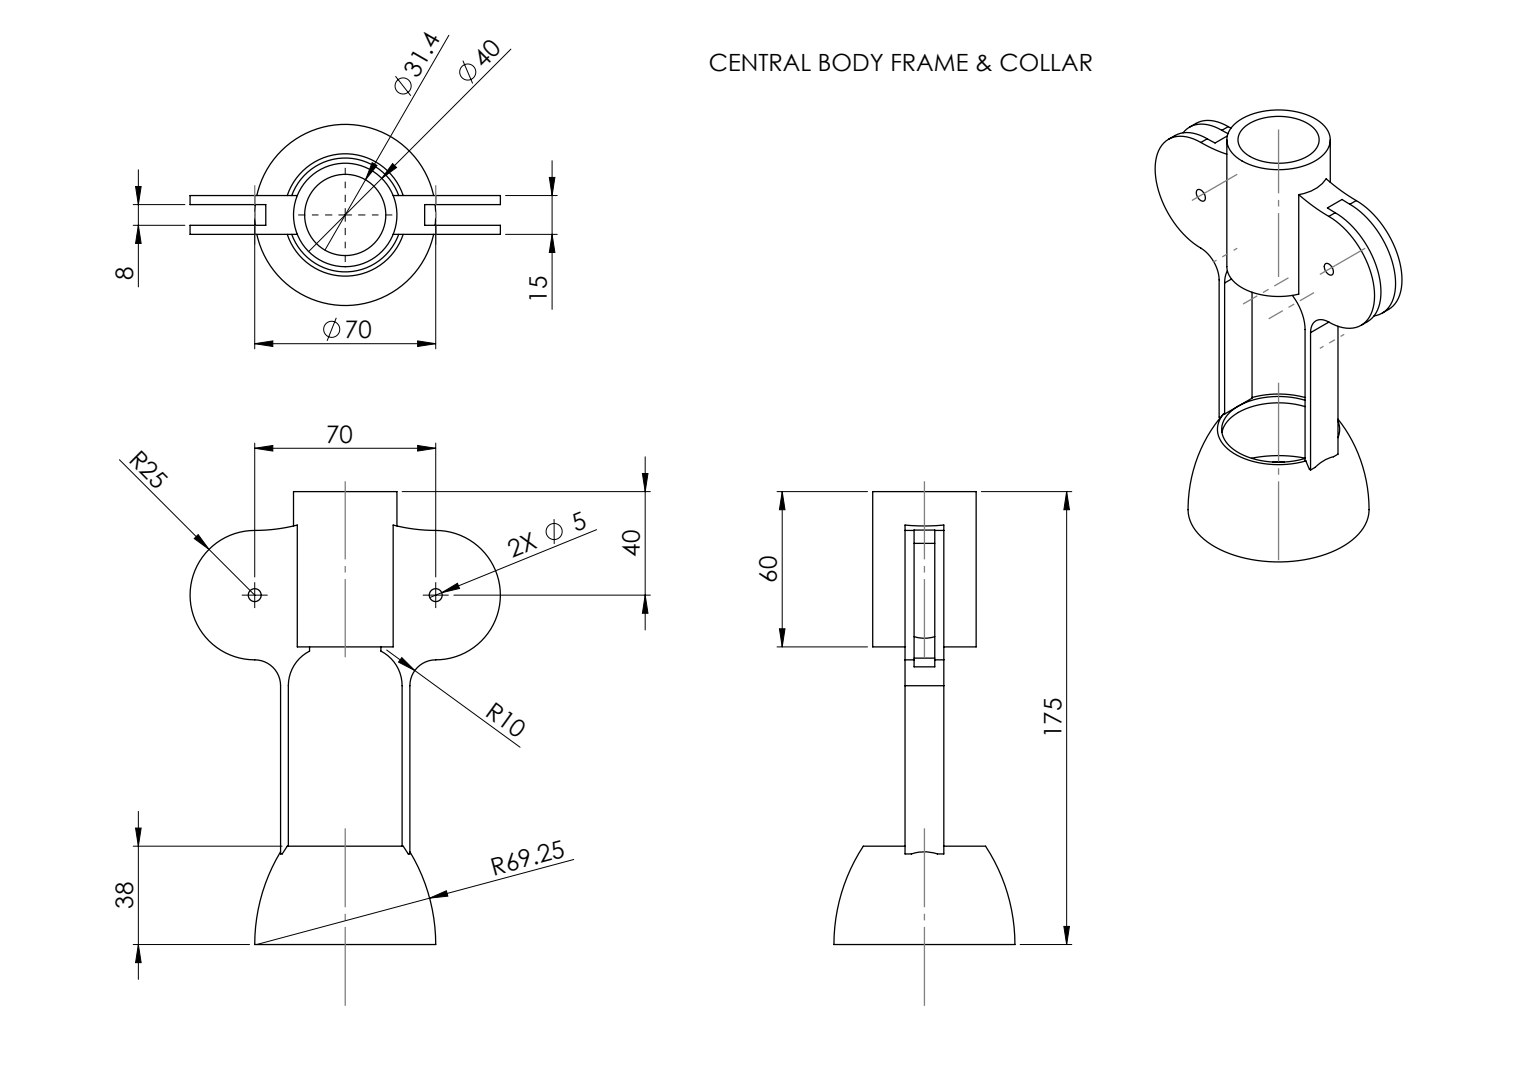
ISO-10303-21;
HEADER;
FILE_DESCRIPTION (('STEP AP214'),
    '1' );
FILE_NAME ('Central Body Frame & Collar.step',
    '2026-10-08T14:03:35',
    ( '' ),
    ( '' ),
    'SwSTEP 2.0',
    'SolidWorks 2026',
    '' );
FILE_SCHEMA (( 'AUTOMOTIVE_DESIGN' ));
ENDSEC;

DATA;
#1=EDGE_LOOP ( 'NONE', ( #6943, #8347, #5492, #144, #24, #10049, #6379, #1001, #2175, #10989 ) ) ;
#8=ORIENTED_EDGE ( 'NONE', *, *, #7820, .F. ) ;
#14=DIRECTION ( 'NONE',  ( -1.000000000000000000, 0.000000000000000000, 0.000000000000000000 ) ) ;
#18=VECTOR ( 'NONE', #6174, 1000.000000000000000 ) ;
#22=ORIENTED_EDGE ( 'NONE', *, *, #10210, .T. ) ;
#24=ORIENTED_EDGE ( 'NONE', *, *, #1458, .F. ) ;
#28=DIRECTION ( 'NONE',  ( -0.000000000000000000, -0.000000000000000000, -1.000000000000000000 ) ) ;
#33=CIRCLE ( 'NONE', #4726, 10.00000000000000178 ) ;
#35=CIRCLE ( 'NONE', #10337, 25.00000000000000711 ) ;
#39=DIRECTION ( 'NONE',  ( 1.000000000000000000, 0.000000000000000000, 0.000000000000000000 ) ) ;
#47=EDGE_LOOP ( 'NONE', ( #4618, #2570, #12122, #10874, #7639, #5291, #7255 ) ) ;
#54=CIRCLE ( 'NONE', #4755, 69.24999999999975842 ) ;
#60=DIRECTION ( 'NONE',  ( -1.000000000000000000, 0.000000000000000000, 0.000000000000000000 ) ) ;
#61=EDGE_CURVE ( 'NONE', #7055, #3214, #4012, .T. ) ;
#65=LINE ( 'NONE', #1951, #2569 ) ;
#67=CARTESIAN_POINT ( 'NONE',  ( -15.18222645069203125, -100.0000000000000000, -4.000000000000000000 ) ) ;
#69=ORIENTED_EDGE ( 'NONE', *, *, #3097, .T. ) ;
#74=ORIENTED_EDGE ( 'NONE', *, *, #8494, .F. ) ;
#75=CARTESIAN_POINT ( 'NONE',  ( -34.99999999999999289, -97.00000000000000000, -7.500000000000000000 ) ) ;
#82=CARTESIAN_POINT ( 'NONE',  ( 25.00000000000001776, -100.0000000000000000, -5.046127144242417373 ) ) ;
#91=ORIENTED_EDGE ( 'NONE', *, *, #2062, .T. ) ;
#97=CARTESIAN_POINT ( 'NONE',  ( -26.79177319725820894, -26.24642857144861807, -4.000000000000000000 ) ) ;
#98=CARTESIAN_POINT ( 'NONE',  ( -60.00000000000001421, -4.286263797015736496E-15, 7.500000000000000000 ) ) ;
#104=CARTESIAN_POINT ( 'NONE',  ( 35.00000000000000000, 4.286263797015736496E-15, 7.500000000000000000 ) ) ;
#107=ORIENTED_EDGE ( 'NONE', *, *, #7623, .T. ) ;
#113=LINE ( 'NONE', #13095, #3464 ) ;
#122=EDGE_CURVE ( 'NONE', #8713, #9553, #6328, .T. ) ;
#123=CARTESIAN_POINT ( 'NONE',  ( 35.00000000000009237, 91.25000000000046896, 4.000000000000000000 ) ) ;
#129=CARTESIAN_POINT ( 'NONE',  ( -35.00000000000000000, -4.286263797015736496E-15, 4.000000000000000000 ) ) ;
#133=EDGE_CURVE ( 'NONE', #3737, #3625, #5810, .T. ) ;
#134=ADVANCED_FACE ( 'NONE', ( #1030, #12741 ), #7261, .F. ) ;
#141=VECTOR ( 'NONE', #5529, 1000.000000000000000 ) ;
#142=CARTESIAN_POINT ( 'NONE',  ( -35.00000000000000000, 25.00000000000000000, -4.000000000000000000 ) ) ;
#144=ORIENTED_EDGE ( 'NONE', *, *, #11064, .F. ) ;
#162=ORIENTED_EDGE ( 'NONE', *, *, #8775, .F. ) ;
#165=FACE_OUTER_BOUND ( 'NONE', #5586, .T. ) ;
#171=DIRECTION ( 'NONE',  ( 0.000000000000000000, 0.000000000000000000, 1.000000000000000000 ) ) ;
#174=CYLINDRICAL_SURFACE ( 'NONE', #4487, 2.500000000000002220 ) ;
#181=DIRECTION ( 'NONE',  ( -0.000000000000000000, -0.000000000000000000, -1.000000000000000000 ) ) ;
#184=CARTESIAN_POINT ( 'NONE',  ( -35.00000000000012079, 91.25000000000045475, -7.500000000000000000 ) ) ;
#194=CARTESIAN_POINT ( 'NONE',  ( 35.00000000000000000, 4.286263797015736496E-15, 4.000000000000000000 ) ) ;
#199=AXIS2_PLACEMENT_3D ( 'NONE', #10505, #5245, #13714 ) ;
#201=AXIS2_PLACEMENT_3D ( 'NONE', #5042, #6172, #12757 ) ;
#202=ORIENTED_EDGE ( 'NONE', *, *, #10624, .T. ) ;
#208=DIRECTION ( 'NONE',  ( 1.000000000000000000, 0.000000000000000000, -0.000000000000000000 ) ) ;
#212=CARTESIAN_POINT ( 'NONE',  ( -13.79311422413708499, -100.0000000000000000, 7.500000000000000000 ) ) ;
#227=AXIS2_PLACEMENT_3D ( 'NONE', #6286, #961, #5222 ) ;
#230=ORIENTED_EDGE ( 'NONE', *, *, #3262, .F. ) ;
#231=DIRECTION ( 'NONE',  ( -1.224646799147353207E-16, 1.000000000000000000, 0.000000000000000000 ) ) ;
#234=DIRECTION ( 'NONE',  ( -1.000000000000000000, 0.000000000000000000, 0.000000000000000000 ) ) ;
#240=CARTESIAN_POINT ( 'NONE',  ( 18.54049621773915746, -20.00000000000000000, -7.500000000000000000 ) ) ;
#249=DIRECTION ( 'NONE',  ( 0.000000000000000000, -1.000000000000000000, 0.000000000000000000 ) ) ;
#253=ORIENTED_EDGE ( 'NONE', *, *, #309, .F. ) ;
#260=DIRECTION ( 'NONE',  ( 0.000000000000000000, 0.000000000000000000, 1.000000000000000000 ) ) ;
#261=FACE_OUTER_BOUND ( 'NONE', #11503, .T. ) ;
#265=ORIENTED_EDGE ( 'NONE', *, *, #867, .T. ) ;
#266=ORIENTED_EDGE ( 'NONE', *, *, #11663, .F. ) ;
#269=EDGE_CURVE ( 'NONE', #10258, #13109, #10073, .T. ) ;
#270=PRODUCT_CONTEXT ( 'NONE', #3147, 'mechanical' ) ;
#276=ADVANCED_FACE ( 'NONE', ( #3756, #3111 ), #953, .F. ) ;
#277=DIRECTION ( 'NONE',  ( -1.000000000000000000, 0.000000000000000000, 0.000000000000000000 ) ) ;
#280=AXIS2_PLACEMENT_3D ( 'NONE', #8444, #12670, #13811 ) ;
#301=EDGE_CURVE ( 'NONE', #2246, #7494, #13812, .T. ) ;
#309=EDGE_CURVE ( 'NONE', #10920, #8708, #4021, .T. ) ;
#324=ORIENTED_EDGE ( 'NONE', *, *, #2209, .F. ) ;
#325=CARTESIAN_POINT ( 'NONE',  ( -22.42156014662057473, -97.00000000000000000, -7.500000000000000000 ) ) ;
#327=CARTESIAN_POINT ( 'NONE',  ( 13.79311422413708499, -20.00000000000000355, 7.500000000000000000 ) ) ;
#328=AXIS2_PLACEMENT_3D ( 'NONE', #13578, #6044, #1960 ) ;
#332=CARTESIAN_POINT ( 'NONE',  ( -19.99988111993867079, 26.72048013816596779, 0.6453928856983819351 ) ) ;
#333=CARTESIAN_POINT ( 'NONE',  ( -35.00000000000000000, -4.286263797015736496E-15, 7.500000000000000000 ) ) ;
#340=ORIENTED_EDGE ( 'NONE', *, *, #4739, .T. ) ;
#345=DIRECTION ( 'NONE',  ( -0.000000000000000000, -0.000000000000000000, -1.000000000000000000 ) ) ;
#348=CARTESIAN_POINT ( 'NONE',  ( -37.50000000000000711, -4.286263797015736496E-15, 7.500000000000000000 ) ) ;
#360=MECHANICAL_DESIGN_GEOMETRIC_PRESENTATION_REPRESENTATION('',(#8623),#10638);
#364=CARTESIAN_POINT ( 'NONE',  ( 19.96844336951937748, 26.72776445485856911, -1.294012040295340782 ) ) ;
#373=ADVANCED_FACE ( 'NONE', ( #13878 ), #5017, .F. ) ;
#376=ORIENTED_EDGE ( 'NONE', *, *, #1897, .T. ) ;
#382=DIRECTION ( 'NONE',  ( 1.000000000000000000, 0.000000000000000000, 0.000000000000000000 ) ) ;
#396=DIRECTION ( 'NONE',  ( -0.000000000000000000, -1.000000000000000000, -0.000000000000000000 ) ) ;
#399=CARTESIAN_POINT ( 'NONE',  ( -13.79311422413708499, -21.62638421600851046, -7.500000000000000000 ) ) ;
#421=LINE ( 'NONE', #1380, #11465 ) ;
#426=FILL_AREA_STYLE ('',( #13278 ) ) ;
#432=ADVANCED_FACE ( 'NONE', ( #819 ), #1931, .T. ) ;
#433=DIRECTION ( 'NONE',  ( -1.000000000000000000, -1.224646799147353207E-16, 0.000000000000000000 ) ) ;
#450=DIRECTION ( 'NONE',  ( -0.000000000000000000, 0.000000000000000000, -1.000000000000000000 ) ) ;
#452=EDGE_CURVE ( 'NONE', #1107, #10314, #12672, .T. ) ;
#457=FACE_OUTER_BOUND ( 'NONE', #1, .T. ) ;
#463=ORIENTED_EDGE ( 'NONE', *, *, #1893, .F. ) ;
#465=CARTESIAN_POINT ( 'NONE',  ( 24.37649275748779232, -100.0000000000000000, -7.500000000000000000 ) ) ;
#466=AXIS2_PLACEMENT_3D ( 'NONE', #1579, #9018, #13326 ) ;
#470=VERTEX_POINT ( 'NONE', #11938 ) ;
#472=VECTOR ( 'NONE', #11869, 1000.000000000000000 ) ;
#473=VECTOR ( 'NONE', #3861, 1000.000000000000000 ) ;
#496=AXIS2_PLACEMENT_3D ( 'NONE', #1680, #5966, #3555 ) ;
#509=DIRECTION ( 'NONE',  ( -1.224646799147353207E-16, 1.000000000000000000, -0.000000000000000000 ) ) ;
#510=CARTESIAN_POINT ( 'NONE',  ( -35.00000000000000000, -20.00000000000000000, 7.500000000000000000 ) ) ;
#521=DIRECTION ( 'NONE',  ( 0.000000000000000000, 0.000000000000000000, 1.000000000000000000 ) ) ;
#524=CARTESIAN_POINT ( 'NONE',  ( -22.00000000000000000, -35.00000000000000000, 7.500000000000000000 ) ) ;
#535=CARTESIAN_POINT ( 'NONE',  ( 18.54049621773915746, -20.00000000000000000, -7.500000000000000000 ) ) ;
#536=ORIENTED_EDGE ( 'NONE', *, *, #1893, .T. ) ;
#540=EDGE_CURVE ( 'NONE', #2953, #6457, #12760, .T. ) ;
#543=EDGE_CURVE ( 'NONE', #5663, #11307, #11801, .T. ) ;
#548=CARTESIAN_POINT ( 'NONE',  ( 35.00000000000000711, -25.00000000000000000, 7.500000000000000000 ) ) ;
#552=CARTESIAN_POINT ( 'NONE',  ( -19.36040733361899768, 26.87219970003945591, -5.058700639371027208 ) ) ;
#557=ORIENTED_EDGE ( 'NONE', *, *, #6920, .T. ) ;
#568=AXIS2_PLACEMENT_3D ( 'NONE', #1899, #1829, #13782 ) ;
#573=EDGE_CURVE ( 'NONE', #11806, #2481, #9618, .T. ) ;
#581=CARTESIAN_POINT ( 'NONE',  ( 19.75162188639114902, 26.77857048203552992, -3.206191164072788702 ) ) ;
#595=DIRECTION ( 'NONE',  ( -1.224646799147353207E-16, 1.000000000000000000, -0.000000000000000000 ) ) ;
#597=CARTESIAN_POINT ( 'NONE',  ( 1.224646799147353217E-14, -100.0000000000000000, 0.000000000000000000 ) ) ;
#598=AXIS2_PLACEMENT_3D ( 'NONE', #9274, #3873, #2045 ) ;
#600=ORIENTED_EDGE ( 'NONE', *, *, #540, .F. ) ;
#604=VECTOR ( 'NONE', #12351, 1000.000000000000000 ) ;
#605=DIRECTION ( 'NONE',  ( 0.000000000000000000, 0.000000000000000000, 1.000000000000000000 ) ) ;
#607=ORIENTED_EDGE ( 'NONE', *, *, #7807, .T. ) ;
#613=FACE_OUTER_BOUND ( 'NONE', #10515, .T. ) ;
#618=VERTEX_POINT ( 'NONE', #399 ) ;
#626=FACE_OUTER_BOUND ( 'NONE', #13070, .T. ) ;
#628=EDGE_CURVE ( 'NONE', #12494, #2284, #10129, .T. ) ;
#635=ADVANCED_FACE ( 'NONE', ( #5923, #12382 ), #2768, .F. ) ;
#640=CARTESIAN_POINT ( 'NONE',  ( -34.99999999999999289, -135.0000000000000000, 0.000000000000000000 ) ) ;
#652=ORIENTED_EDGE ( 'NONE', *, *, #5322, .F. ) ;
#659=ORIENTED_EDGE ( 'NONE', *, *, #7380, .T. ) ;
#661=ORIENTED_EDGE ( 'NONE', *, *, #10607, .F. ) ;
#665=ORIENTED_EDGE ( 'NONE', *, *, #2832, .F. ) ;
#681=AXIS2_PLACEMENT_3D ( 'NONE', #12169, #3822, #11262 ) ;
#685=ORIENTED_EDGE ( 'NONE', *, *, #12001, .T. ) ;
#690=CARTESIAN_POINT ( 'NONE',  ( 0.000000000000000000, 0.000000000000000000, 0.000000000000000000 ) ) ;
#697=VECTOR ( 'NONE', #5522, 1000.000000000000000 ) ;
#709=CARTESIAN_POINT ( 'NONE',  ( -25.00000000000000000, -35.00000000000000000, 7.500000000000000000 ) ) ;
#711=DIRECTION ( 'NONE',  ( 0.000000000000000000, 1.000000000000000000, 0.000000000000000000 ) ) ;
#716=ORIENTED_EDGE ( 'NONE', *, *, #10582, .F. ) ;
#719=EDGE_CURVE ( 'NONE', #13879, #9113, #9755, .T. ) ;
#728=CARTESIAN_POINT ( 'NONE',  ( -14.41066181492265308, -21.94006687227777874, -6.364279405527200062 ) ) ;
#733=EDGE_LOOP ( 'NONE', ( #2396, #11229, #1811, #8877, #4164, #2069 ) ) ;
#737=VECTOR ( 'NONE', #6051, 1000.000000000000000 ) ;
#742=CARTESIAN_POINT ( 'NONE',  ( -35.00000000000000000, -4.286263797015736496E-15, -4.000000000000000000 ) ) ;
#764=CARTESIAN_POINT ( 'NONE',  ( -35.00000000000000711, -25.00000000000000711, 4.000000000000000000 ) ) ;
#766=VECTOR ( 'NONE', #12559, 1000.000000000000000 ) ;
#767=ORIENTED_EDGE ( 'NONE', *, *, #13181, .F. ) ;
#774=LINE ( 'NONE', #6035, #604 ) ;
#777=CARTESIAN_POINT ( 'NONE',  ( -35.00000000000000000, -35.00000000000000000, -7.500000000000000000 ) ) ;
#792=EDGE_CURVE ( 'NONE', #6662, #8229, #1784, .T. ) ;
#799=AXIS2_PLACEMENT_3D ( 'NONE', #2482, #11030, #5781 ) ;
#801=EDGE_CURVE ( 'NONE', #3433, #1175, #9060, .T. ) ;
#806=CARTESIAN_POINT ( 'NONE',  ( 37.50000000000000711, 4.592425496802575156E-15, 7.500000000000000000 ) ) ;
#809=DIRECTION ( 'NONE',  ( -1.224646799147353207E-16, -1.499759782661857608E-32, 1.000000000000000000 ) ) ;
#812=AXIS2_PLACEMENT_3D ( 'NONE', #11782, #8689, #9817 ) ;
#819=FACE_OUTER_BOUND ( 'NONE', #8492, .T. ) ;
#827=FACE_OUTER_BOUND ( 'NONE', #12015, .T. ) ;
#836=ORIENTED_EDGE ( 'NONE', *, *, #122, .F. ) ;
#841=LINE ( 'NONE', #11493, #7119 ) ;
#847=ORIENTED_EDGE ( 'NONE', *, *, #3025, .F. ) ;
#866=AXIS2_PLACEMENT_3D ( 'NONE', #6033, #509, #433 ) ;
#867=EDGE_CURVE ( 'NONE', #11483, #10241, #6721, .T. ) ;
#871=CARTESIAN_POINT ( 'NONE',  ( -25.00000000000000000, -35.00000000000000000, -7.500000000000000000 ) ) ;
#877=DIRECTION ( 'NONE',  ( 1.000000000000000000, 0.000000000000000000, 0.000000000000000000 ) ) ;
#896=VECTOR ( 'NONE', #3103, 1000.000000000000000 ) ;
#898=AXIS2_PLACEMENT_3D ( 'NONE', #3051, #9567, #7189 ) ;
#903=CARTESIAN_POINT ( 'NONE',  ( 32.50000000000000000, 4.286263797015736496E-15, -7.500000000000000000 ) ) ;
#907=DIRECTION ( 'NONE',  ( 0.000000000000000000, 0.000000000000000000, 1.000000000000000000 ) ) ;
#914=EDGE_LOOP ( 'NONE', ( #376, #7478 ) ) ;
#915=CIRCLE ( 'NONE', #1137, 31.93204061526060755 ) ;
#916=DIRECTION ( 'NONE',  ( -1.000000000000000000, 0.000000000000000000, 0.000000000000000000 ) ) ;
#919=B_SPLINE_CURVE_WITH_KNOTS ( 'NONE', 3,
 ( #9871, #5582, #12906, #4525, #4389, #3338, #10902, #2151 ),
 .UNSPECIFIED., .F., .F.,
 ( 4, 2, 2, 4 ),
 ( 0.02189346042269462930, 0.02442701477284300177, 0.02569379194791718973, 0.02696056912299137770 ),
 .UNSPECIFIED. ) ;
#927=CIRCLE ( 'NONE', #10546, 21.99999999999999289 ) ;
#932=CARTESIAN_POINT ( 'NONE',  ( 1.653273178848927024E-14, -135.0000000000000000, 0.000000000000000000 ) ) ;
#934=EDGE_LOOP ( 'NONE', ( #5830, #10072 ) ) ;
#939=DIRECTION ( 'NONE',  ( 1.000000000000000000, 0.000000000000000000, 0.000000000000000000 ) ) ;
#948=DIRECTION ( 'NONE',  ( -1.000000000000000000, 0.000000000000000000, 0.000000000000000000 ) ) ;
#953=PLANE ( 'NONE',  #898 ) ;
#961=DIRECTION ( 'NONE',  ( -0.000000000000000000, 0.000000000000000000, -1.000000000000000000 ) ) ;
#966=EDGE_CURVE ( 'NONE', #3769, #3176, #4398, .T. ) ;
#975=DIRECTION ( 'NONE',  ( 1.000000000000000000, 1.224646799147353207E-16, 0.000000000000000000 ) ) ;
#979=EDGE_CURVE ( 'NONE', #4467, #10258, #13122, .T. ) ;
#985=FACE_OUTER_BOUND ( 'NONE', #11435, .T. ) ;
#986=ORIENTED_EDGE ( 'NONE', *, *, #8544, .T. ) ;
#998=DIRECTION ( 'NONE',  ( -1.000000000000000000, 0.000000000000000000, 0.000000000000000000 ) ) ;
#1000=ORIENTED_EDGE ( 'NONE', *, *, #11502, .T. ) ;
#1001=ORIENTED_EDGE ( 'NONE', *, *, #13764, .T. ) ;
#1002=AXIS2_PLACEMENT_3D ( 'NONE', #11272, #5952, #10357 ) ;
#1004=ORIENTED_EDGE ( 'NONE', *, *, #10303, .F. ) ;
#1017=CARTESIAN_POINT ( 'NONE',  ( 34.24999999999975842, -135.0000000000000000, 0.000000000000000000 ) ) ;
#1018=CARTESIAN_POINT ( 'NONE',  ( -28.79177319725820894, -26.24642857144861807, -4.000000000000000000 ) ) ;
#1030=FACE_BOUND ( 'NONE', #4686, .T. ) ;
#1034=AXIS2_PLACEMENT_3D ( 'NONE', #5912, #7786, #12369 ) ;
#1043=ORIENTED_EDGE ( 'NONE', *, *, #4815, .T. ) ;
#1053=FACE_OUTER_BOUND ( 'NONE', #11895, .T. ) ;
#1059=ORIENTED_EDGE ( 'NONE', *, *, #4359, .T. ) ;
#1061=CARTESIAN_POINT ( 'NONE',  ( -60.00000000000001421, 20.00000000000000000, 4.000000000000000000 ) ) ;
#1066=DIRECTION ( 'NONE',  ( -1.000000000000000000, 0.000000000000000000, 0.000000000000000000 ) ) ;
#1073=DIRECTION ( 'NONE',  ( -1.000000000000000000, 0.000000000000000000, 0.000000000000000000 ) ) ;
#1077=DIRECTION ( 'NONE',  ( -1.224646799147353207E-16, 1.000000000000000000, -0.000000000000000000 ) ) ;
#1082=EDGE_CURVE ( 'NONE', #6722, #11449, #5669, .T. ) ;
#1092=ORIENTED_EDGE ( 'NONE', *, *, #61, .F. ) ;
#1093=CARTESIAN_POINT ( 'NONE',  ( -32.50000000000000000, -3.980102097228898626E-15, -4.000000000000000000 ) ) ;
#1097=AXIS2_PLACEMENT_3D ( 'NONE', #9065, #13450, #4710 ) ;
#1107=VERTEX_POINT ( 'NONE', #3516 ) ;
#1113=DIRECTION ( 'NONE',  ( -0.000000000000000000, -0.000000000000000000, -1.000000000000000000 ) ) ;
#1121=AXIS2_PLACEMENT_3D ( 'NONE', #5344, #1273, #9629 ) ;
#1123=ADVANCED_FACE ( 'NONE', ( #3312 ), #7797, .F. ) ;
#1134=LINE ( 'NONE', #8488, #10413 ) ;
#1137=AXIS2_PLACEMENT_3D ( 'NONE', #9842, #9775, #5630 ) ;
#1138=ORIENTED_EDGE ( 'NONE', *, *, #7758, .T. ) ;
#1140=ORIENTED_EDGE ( 'NONE', *, *, #4608, .F. ) ;
#1142=ADVANCED_FACE ( 'NONE', ( #12014 ), #6615, .F. ) ;
#1150=CIRCLE ( 'NONE', #496, 20.00000000000000000 ) ;
#1151=DIRECTION ( 'NONE',  ( 0.000000000000000000, 1.000000000000000000, 0.000000000000000000 ) ) ;
#1156=DIRECTION ( 'NONE',  ( -1.000000000000000000, 0.000000000000000000, 0.000000000000000000 ) ) ;
#1162=DIRECTION ( 'NONE',  ( -1.000000000000000000, 0.000000000000000000, 0.000000000000000000 ) ) ;
#1164=EDGE_LOOP ( 'NONE', ( #8091, #8679, #11162, #3980 ) ) ;
#1169=LINE ( 'NONE', #9923, #5204 ) ;
#1175=VERTEX_POINT ( 'NONE', #6831 ) ;
#1182=CARTESIAN_POINT ( 'NONE',  ( 23.75221630157310315, -98.98132178242397572, 7.500000000000000000 ) ) ;
#1184=EDGE_LOOP ( 'NONE', ( #6080, #7628, #1059, #324 ) ) ;
#1192=DIRECTION ( 'NONE',  ( 2.668805347656626185E-16, -1.000000000000000000, -0.000000000000000000 ) ) ;
#1195=CARTESIAN_POINT ( 'NONE',  ( -24.99999999999999289, -99.86284836912238916, 4.640101051368102247 ) ) ;
#1207=( NAMED_UNIT ( * ) PLANE_ANGLE_UNIT ( ) SI_UNIT ( $, .RADIAN. ) );
#1214=EDGE_CURVE ( 'NONE', #4795, #6682, #915, .T. ) ;
#1218=DIRECTION ( 'NONE',  ( 0.000000000000000000, 1.000000000000000000, 0.000000000000000000 ) ) ;
#1223=VECTOR ( 'NONE', #10636, 1000.000000000000000 ) ;
#1254=EDGE_LOOP ( 'NONE', ( #12301, #6976, #1516, #6221, #12477, #13271, #4805, #4411 ) ) ;
#1258=CARTESIAN_POINT ( 'NONE',  ( -18.54049621773915746, -20.00000000000000000, -7.500000000000000000 ) ) ;
#1259=DIRECTION ( 'NONE',  ( -1.000000000000000000, 0.000000000000000000, 0.000000000000000000 ) ) ;
#1263=DIRECTION ( 'NONE',  ( -0.000000000000000000, -0.000000000000000000, -1.000000000000000000 ) ) ;
#1266=CIRCLE ( 'NONE', #10884, 10.00000000000000178 ) ;
#1273=DIRECTION ( 'NONE',  ( -0.000000000000000000, -0.000000000000000000, -1.000000000000000000 ) ) ;
#1275=FACE_OUTER_BOUND ( 'NONE', #7688, .T. ) ;
#1276=DIRECTION ( 'NONE',  ( -1.000000000000000000, 0.000000000000000000, 0.000000000000000000 ) ) ;
#1280=DIRECTION ( 'NONE',  ( -1.000000000000000000, 0.000000000000000000, 0.000000000000000000 ) ) ;
#1285=CARTESIAN_POINT ( 'NONE',  ( -24.99999999999999645, -99.15310334213022259, -0.4257687054510825297 ) ) ;
#1288=ORIENTED_EDGE ( 'NONE', *, *, #12701, .F. ) ;
#1292=DIRECTION ( 'NONE',  ( -0.000000000000000000, -0.000000000000000000, -1.000000000000000000 ) ) ;
#1300=DIRECTION ( 'NONE',  ( -0.000000000000000000, -0.000000000000000000, -1.000000000000000000 ) ) ;
#1301=CIRCLE ( 'NONE', #4422, 15.70031846811053455 ) ;
#1305=ORIENTED_EDGE ( 'NONE', *, *, #1729, .F. ) ;
#1318=FACE_BOUND ( 'NONE', #1621, .T. ) ;
#1330=ORIENTED_EDGE ( 'NONE', *, *, #1895, .T. ) ;
#1332=( NAMED_UNIT ( * ) PLANE_ANGLE_UNIT ( ) SI_UNIT ( $, .RADIAN. ) );
#1335=VECTOR ( 'NONE', #12650, 1000.000000000000000 ) ;
#1343=ORIENTED_EDGE ( 'NONE', *, *, #7796, .T. ) ;
#1348=FACE_BOUND ( 'NONE', #3706, .T. ) ;
#1349=CIRCLE ( 'NONE', #3140, 25.50418395392908977 ) ;
#1355=VERTEX_POINT ( 'NONE', #1774 ) ;
#1372=ORIENTED_EDGE ( 'NONE', *, *, #3276, .F. ) ;
#1380=CARTESIAN_POINT ( 'NONE',  ( -37.50000000000000711, -4.286263797015736496E-15, 7.500000000000000000 ) ) ;
#1381=DIRECTION ( 'NONE',  ( 1.000000000000000000, 0.000000000000000000, 0.000000000000000000 ) ) ;
#1387=PRODUCT ( 'Central Body Frame & Collar', 'Central Body Frame & Collar', '', ( #270 ) ) ;
#1390=ORIENTED_EDGE ( 'NONE', *, *, #7706, .F. ) ;
#1392=DIRECTION ( 'NONE',  ( 1.000000000000000000, 6.938893903907227392E-16, 0.000000000000000000 ) ) ;
#1399=CARTESIAN_POINT ( 'NONE',  ( 22.00000000000000355, -34.99999999999999289, 7.500000000000000000 ) ) ;
#1407=VERTEX_POINT ( 'NONE', #7746 ) ;
#1409=CARTESIAN_POINT ( 'NONE',  ( 0.000000000000000000, 0.000000000000000000, 0.000000000000000000 ) ) ;
#1420=AXIS2_PLACEMENT_3D ( 'NONE', #4195, #5059, #13652 ) ;
#1423=CIRCLE ( 'NONE', #7924, 10.00000000000000178 ) ;
#1458=EDGE_CURVE ( 'NONE', #9642, #2246, #1349, .T. ) ;
#1464=AXIS2_PLACEMENT_3D ( 'NONE', #932, #5068, #998 ) ;
#1465=EDGE_CURVE ( 'NONE', #3209, #7690, #13263, .T. ) ;
#1480=FILL_AREA_STYLE ('',( #4347 ) ) ;
#1488=CARTESIAN_POINT ( 'NONE',  ( 15.18222645069203303, -16.04698886238941924, 4.000000000000000000 ) ) ;
#1500=FACE_OUTER_BOUND ( 'NONE', #11636, .T. ) ;
#1502=CARTESIAN_POINT ( 'NONE',  ( 22.42156014662059249, -97.00000000000000000, 7.500000000000000000 ) ) ;
#1506=DIRECTION ( 'NONE',  ( 0.000000000000000000, 0.000000000000000000, 1.000000000000000000 ) ) ;
#1516=ORIENTED_EDGE ( 'NONE', *, *, #7775, .T. ) ;
#1534=DIRECTION ( 'NONE',  ( 1.000000000000000000, 0.000000000000000000, 0.000000000000000000 ) ) ;
#1545=VERTEX_POINT ( 'NONE', #8855 ) ;
#1547=CARTESIAN_POINT ( 'NONE',  ( -23.75056915604791286, -98.97863401284405427, 7.500000000000000000 ) ) ;
#1551=B_SPLINE_CURVE_WITH_KNOTS ( 'NONE', 3,
 ( #7248, #5282, #11532, #9365, #1925, #6213, #6407, #10608 ),
 .UNSPECIFIED., .F., .F.,
 ( 4, 2, 2, 4 ),
 ( 0.02696056912299137770, 0.02949568642151915651, 0.03076324507078304765, 0.03203080372004693532 ),
 .UNSPECIFIED. ) ;
#1560=ORIENTED_EDGE ( 'NONE', *, *, #3191, .F. ) ;
#1563=ADVANCED_FACE ( 'NONE', ( #1348, #3447 ), #9839, .F. ) ;
#1573=ORIENTED_EDGE ( 'NONE', *, *, #5943, .T. ) ;
#1578=CARTESIAN_POINT ( 'NONE',  ( 1.387778780781445676E-14, -135.0000000000000000, 0.000000000000000000 ) ) ;
#1579=CARTESIAN_POINT ( 'NONE',  ( 35.00000000000000000, 4.286263797015736496E-15, 7.500000000000000000 ) ) ;
#1592=VERTEX_POINT ( 'NONE', #5777 ) ;
#1593=DIRECTION ( 'NONE',  ( 0.000000000000000000, 1.000000000000000000, 0.000000000000000000 ) ) ;
#1594=CARTESIAN_POINT ( 'NONE',  ( -24.99999999999998934, -100.0000000000000000, 7.500000000000000000 ) ) ;
#1605=EDGE_LOOP ( 'NONE', ( #2349, #69, #5334, #6879, #8263, #11647 ) ) ;
#1612=MECHANICAL_DESIGN_GEOMETRIC_PRESENTATION_REPRESENTATION('',(#10127),#11476);
#1617=ORIENTED_EDGE ( 'NONE', *, *, #2561, .T. ) ;
#1621=EDGE_LOOP ( 'NONE', ( #13498, #11507 ) ) ;
#1625=DIRECTION ( 'NONE',  ( -1.000000000000000000, 0.000000000000000000, 0.000000000000000000 ) ) ;
#1639=EDGE_CURVE ( 'NONE', #5724, #13483, #3153, .T. ) ;
#1640=DIRECTION ( 'NONE',  ( -1.000000000000000000, 0.000000000000000000, 0.000000000000000000 ) ) ;
#1651=LINE ( 'NONE', #548, #1823 ) ;
#1653=CARTESIAN_POINT ( 'NONE',  ( -6.999999999999999112, -20.00000000000000355, 7.500000000000000000 ) ) ;
#1657=CARTESIAN_POINT ( 'NONE',  ( -18.54049621773915746, 27.07720798311999388, -7.500000000000000000 ) ) ;
#1672=CARTESIAN_POINT ( 'NONE',  ( -15.18222645069203303, -16.04698886238941924, 4.000000000000000000 ) ) ;
#1680=CARTESIAN_POINT ( 'NONE',  ( 0.000000000000000000, 40.00000000000000000, 0.000000000000000000 ) ) ;
#1684=CARTESIAN_POINT ( 'NONE',  ( 18.54049621773915746, 27.07720798312000809, -7.500000000000000000 ) ) ;
#1698=CIRCLE ( 'NONE', #9311, 66.25000000000044054 ) ;
#1708=FACE_OUTER_BOUND ( 'NONE', #10037, .T. ) ;
#1721=VECTOR ( 'NONE', #11277, 1000.000000000000000 ) ;
#1729=EDGE_CURVE ( 'NONE', #5794, #3209, #35, .T. ) ;
#1742=EDGE_CURVE ( 'NONE', #10695, #7989, #11835, .T. ) ;
#1755=CYLINDRICAL_SURFACE ( 'NONE', #568, 2.500000000000002220 ) ;
#1760=CIRCLE ( 'NONE', #10277, 66.25000000000044054 ) ;
#1761=CARTESIAN_POINT ( 'NONE',  ( -25.00000000000000000, -35.00000000000000000, 7.500000000000000000 ) ) ;
#1763=CARTESIAN_POINT ( 'NONE',  ( 26.79177319725820539, -26.24642857144861807, -4.000000000000000000 ) ) ;
#1765=CARTESIAN_POINT ( 'NONE',  ( 28.79177319725820183, -26.24642857144861807, 4.000000000000000000 ) ) ;
#1767=ORIENTED_EDGE ( 'NONE', *, *, #13765, .T. ) ;
#1769=ORIENTED_EDGE ( 'NONE', *, *, #10970, .T. ) ;
#1773=CARTESIAN_POINT ( 'NONE',  ( -34.99999999999999289, -97.00000000000000000, 7.500000000000000000 ) ) ;
#1774=CARTESIAN_POINT ( 'NONE',  ( -35.00000000000000711, -25.00000000000000711, -4.000000000000000000 ) ) ;
#1775=DIRECTION ( 'NONE',  ( -1.000000000000000000, 0.000000000000000000, 0.000000000000000000 ) ) ;
#1778=DIRECTION ( 'NONE',  ( -1.224646799147353207E-16, 1.000000000000000000, -0.000000000000000000 ) ) ;
#1784=B_SPLINE_CURVE_WITH_KNOTS ( 'NONE', 3,
 ( #5981, #1547, #2676, #4703 ),
 .UNSPECIFIED., .F., .F.,
 ( 4, 4 ),
 ( 0.02301878569831470461, 0.02656428146801016396 ),
 .UNSPECIFIED. ) ;
#1810=AXIS2_PLACEMENT_3D ( 'NONE', #8096, #7036, #6971 ) ;
#1811=ORIENTED_EDGE ( 'NONE', *, *, #6765, .F. ) ;
#1823=VECTOR ( 'NONE', #1850, 1000.000000000000000 ) ;
#1824=AXIS2_PLACEMENT_3D ( 'NONE', #8707, #9911, #1280 ) ;
#1829=DIRECTION ( 'NONE',  ( -0.000000000000000000, -0.000000000000000000, -1.000000000000000000 ) ) ;
#1837=CARTESIAN_POINT ( 'NONE',  ( -15.04986406078725203, -22.34153611474686940, 4.519294538364308167 ) ) ;
#1839=DIRECTION ( 'NONE',  ( -0.000000000000000000, -0.000000000000000000, -1.000000000000000000 ) ) ;
#1850=DIRECTION ( 'NONE',  ( -0.000000000000000000, -0.000000000000000000, -1.000000000000000000 ) ) ;
#1855=ADVANCED_FACE ( 'NONE', ( #11348 ), #10367, .F. ) ;
#1857=ORIENTED_EDGE ( 'NONE', *, *, #573, .T. ) ;
#1862=CIRCLE ( 'NONE', #4780, 1.999999999999998224 ) ;
#1867=AXIS2_PLACEMENT_3D ( 'NONE', #4523, #9939, #6567 ) ;
#1868=CARTESIAN_POINT ( 'NONE',  ( -15.48128881649354405, -16.40999965198128052, 2.699219240941213460 ) ) ;
#1873=DIRECTION ( 'NONE',  ( -1.000000000000000000, 0.000000000000000000, 0.000000000000000000 ) ) ;
#1881=DIRECTION ( 'NONE',  ( -1.224646799147353207E-16, 1.000000000000000000, -0.000000000000000000 ) ) ;
#1882=CARTESIAN_POINT ( 'NONE',  ( -24.99999999999998934, -99.15310334213020838, 4.530792947966844994E-20 ) ) ;
#1883=DIRECTION ( 'NONE',  ( -0.000000000000000000, -0.000000000000000000, -1.000000000000000000 ) ) ;
#1891=EDGE_CURVE ( 'NONE', #3176, #9535, #2765, .T. ) ;
#1893=EDGE_CURVE ( 'NONE', #13392, #7522, #6891, .T. ) ;
#1895=EDGE_CURVE ( 'NONE', #5016, #8361, #13461, .T. ) ;
#1897=EDGE_CURVE ( 'NONE', #3490, #7522, #2043, .T. ) ;
#1899=CARTESIAN_POINT ( 'NONE',  ( 35.00000000000000000, 4.286263797015736496E-15, 7.500000000000000000 ) ) ;
#1912=AXIS2_PLACEMENT_3D ( 'NONE', #6617, #9993, #3453 ) ;
#1916=CIRCLE ( 'NONE', #9977, 25.50000000002550138 ) ;
#1921=DIRECTION ( 'NONE',  ( -1.000000000000000000, 0.000000000000000000, 0.000000000000000000 ) ) ;
#1922=CIRCLE ( 'NONE', #6395, 66.25000000000044054 ) ;
#1925=CARTESIAN_POINT ( 'NONE',  ( 25.00000000000001776, -99.52837026979787538, -3.391106264173641804 ) ) ;
#1926=CARTESIAN_POINT ( 'NONE',  ( -35.00000000000000000, -4.286263797015736496E-15, -4.000000000000000000 ) ) ;
#1931=CYLINDRICAL_SURFACE ( 'NONE', #12325, 20.00000000000000000 ) ;
#1935=ADVANCED_FACE ( 'NONE', ( #1708 ), #11103, .F. ) ;
#1946=VECTOR ( 'NONE', #3403, 1000.000000000000000 ) ;
#1947=VERTEX_POINT ( 'NONE', #13237 ) ;
#1951=CARTESIAN_POINT ( 'NONE',  ( -34.99999999999999289, -97.00000000000000000, 7.500000000000000000 ) ) ;
#1953=DIRECTION ( 'NONE',  ( -1.000000000000000000, 0.000000000000000000, 0.000000000000000000 ) ) ;
#1954=DIRECTION ( 'NONE',  ( 0.000000000000000000, -1.000000000000000000, 0.000000000000000000 ) ) ;
#1960=DIRECTION ( 'NONE',  ( -1.000000000000000000, -1.224646799147353207E-16, 0.000000000000000000 ) ) ;
#1962=ORIENTED_EDGE ( 'NONE', *, *, #10232, .F. ) ;
#1968=EDGE_CURVE ( 'NONE', #6184, #2827, #6710, .T. ) ;
#1969=CARTESIAN_POINT ( 'NONE',  ( 25.00000000000001421, -34.99999999999999289, 7.500000000000000000 ) ) ;
#1971=DIRECTION ( 'NONE',  ( -1.000000000000000000, 0.000000000000000000, 0.000000000000000000 ) ) ;
#2001=AXIS2_PLACEMENT_3D ( 'NONE', #7506, #28, #9822 ) ;
#2004=CARTESIAN_POINT ( 'NONE',  ( 32.50000000000000000, 4.286263797015736496E-15, 4.000000000000000000 ) ) ;
#2005=CLOSED_SHELL ( 'NONE', ( #4581, #9687, #11319, #9460, #3588, #10218, #432, #8396, #12006, #5588, #1563, #10694, #6032, #9638, #13585, #7458, #2471, #10229, #10027, #9796, #11511, #11935, #7208, #3950, #13273, #1123, #134, #12776, #635, #4031, #7282, #4048, #1855, #1935, #7213, #1142, #11590, #373, #8410, #7642, #10385, #2232, #9948, #11328, #12394, #6267, #11141, #2908, #12565, #9946, #4471, #7700, #5610, #12266, #276, #9178, #10300, #11770, #8830, #5086, #5399, #3266, #9691, #8262 ) ) ;
#2006=CARTESIAN_POINT ( 'NONE',  ( 15.70089697932620609, -22.78139155752743861, -0.6412871628180832895 ) ) ;
#2015=EDGE_LOOP ( 'NONE', ( #12881, #12979, #6300, #7435 ) ) ;
#2023=DIRECTION ( 'NONE',  ( 1.000000000000000000, 0.000000000000000000, 0.000000000000000000 ) ) ;
#2024=ORIENTED_EDGE ( 'NONE', *, *, #5099, .T. ) ;
#2042=CARTESIAN_POINT ( 'NONE',  ( 0.000000000000000000, -20.00000000000000355, 0.000000000000000000 ) ) ;
#2043=CIRCLE ( 'NONE', #13515, 2.500000000000002220 ) ;
#2045=DIRECTION ( 'NONE',  ( 1.000000000000000000, 0.000000000000000000, 0.000000000000000000 ) ) ;
#2046=EDGE_LOOP ( 'NONE', ( #2111, #2784, #3306, #10881 ) ) ;
#2052=ORIENTED_EDGE ( 'NONE', *, *, #10986, .T. ) ;
#2062=EDGE_CURVE ( 'NONE', #1545, #10464, #6058, .T. ) ;
#2063=B_SPLINE_CURVE_WITH_KNOTS ( 'NONE', 3,
 ( #8757, #9610, #10590, #12780, #3151, #7357, #1195, #4201 ),
 .UNSPECIFIED., .F., .F.,
 ( 4, 2, 2, 4 ),
 ( 0.02696056912299139158, 0.02949568642151887896, 0.03076324507078262438, 0.03203080372004636633 ),
 .UNSPECIFIED. ) ;
#2069=ORIENTED_EDGE ( 'NONE', *, *, #6685, .F. ) ;
#2072=DIRECTION ( 'NONE',  ( 0.000000000000000000, 1.000000000000000000, -0.000000000000000000 ) ) ;
#2085=LINE ( 'NONE', #11621, #5695 ) ;
#2092=ORIENTED_EDGE ( 'NONE', *, *, #1968, .F. ) ;
#2094=EDGE_CURVE ( 'NONE', #8094, #6099, #10548, .T. ) ;
#2095=DIRECTION ( 'NONE',  ( -0.000000000000000000, -0.000000000000000000, -1.000000000000000000 ) ) ;
#2103=DIRECTION ( 'NONE',  ( 2.668805347656626185E-16, -1.000000000000000000, -0.000000000000000000 ) ) ;
#2107=ORIENTED_EDGE ( 'NONE', *, *, #792, .F. ) ;
#2111=ORIENTED_EDGE ( 'NONE', *, *, #12193, .F. ) ;
#2130=CARTESIAN_POINT ( 'NONE',  ( 25.00000000000001776, -100.0000000000000000, 7.500000000000000000 ) ) ;
#2131=AXIS2_PLACEMENT_3D ( 'NONE', #597, #13456, #6198 ) ;
#2136=CARTESIAN_POINT ( 'NONE',  ( -26.79177319725820894, -26.24642857144861807, 4.000000000000000000 ) ) ;
#2140=CARTESIAN_POINT ( 'NONE',  ( -35.00000000000000000, -4.286263797015736496E-15, 7.500000000000000000 ) ) ;
#2144=EDGE_CURVE ( 'NONE', #7494, #9642, #5149, .T. ) ;
#2146=VECTOR ( 'NONE', #7472, 1000.000000000000000 ) ;
#2151=CARTESIAN_POINT ( 'NONE',  ( 25.00000000000001776, -99.15310334213020838, 3.061571689641656246E-15 ) ) ;
#2153=CARTESIAN_POINT ( 'NONE',  ( -21.99999999999999289, -97.00000000000000000, 0.000000000000000000 ) ) ;
#2157=ORIENTED_EDGE ( 'NONE', *, *, #12861, .T. ) ;
#2163=ORIENTED_EDGE ( 'NONE', *, *, #10211, .T. ) ;
#2166=EDGE_CURVE ( 'NONE', #6722, #5663, #7164, .T. ) ;
#2167=DIRECTION ( 'NONE',  ( 0.000000000000000000, 0.000000000000000000, 1.000000000000000000 ) ) ;
#2169=LINE ( 'NONE', #8107, #10901 ) ;
#2171=DIRECTION ( 'NONE',  ( -1.000000000000000000, 0.000000000000000000, 0.000000000000000000 ) ) ;
#2175=ORIENTED_EDGE ( 'NONE', *, *, #10365, .F. ) ;
#2182=CARTESIAN_POINT ( 'NONE',  ( 25.00000000000001776, -100.0000000000000000, 7.500000000000000000 ) ) ;
#2190=AXIS2_PLACEMENT_3D ( 'NONE', #2235, #2298, #1259 ) ;
#2191=DIRECTION ( 'NONE',  ( 1.000000000000000000, 0.000000000000000000, 0.000000000000000000 ) ) ;
#2197=LINE ( 'NONE', #5423, #2572 ) ;
#2206=DIRECTION ( 'NONE',  ( 1.000000000000000000, 0.000000000000000000, 0.000000000000000000 ) ) ;
#2209=EDGE_CURVE ( 'NONE', #12961, #5520, #5627, .T. ) ;
#2216=AXIS2_PLACEMENT_3D ( 'NONE', #5831, #8078, #13521 ) ;
#2219=CARTESIAN_POINT ( 'NONE',  ( -35.00000000000000000, -4.286263797015736496E-15, -4.000000000000000000 ) ) ;
#2231=ORIENTED_EDGE ( 'NONE', *, *, #13332, .T. ) ;
#2232=ADVANCED_FACE ( 'NONE', ( #8780 ), #11937, .F. ) ;
#2235=CARTESIAN_POINT ( 'NONE',  ( 1.187907395172932673E-14, -97.00000000000000000, 0.000000000000000000 ) ) ;
#2241=FACE_OUTER_BOUND ( 'NONE', #3052, .T. ) ;
#2242=ORIENTED_EDGE ( 'NONE', *, *, #4739, .F. ) ;
#2246=VERTEX_POINT ( 'NONE', #7586 ) ;
#2250=ORIENTED_EDGE ( 'NONE', *, *, #801, .F. ) ;
#2256=VECTOR ( 'NONE', #396, 1000.000000000000000 ) ;
#2257=DIRECTION ( 'NONE',  ( 0.000000000000000000, 1.000000000000000000, -0.000000000000000000 ) ) ;
#2260=B_SPLINE_CURVE_WITH_KNOTS ( 'NONE', 3,
 ( #2790, #7194, #4885, #10424, #9164, #13489, #9240, #12402, #11475, #1868, #10286, #5025 ),
 .UNSPECIFIED., .F., .F.,
 ( 4, 2, 2, 2, 2, 4 ),
 ( 0.000000000000000000, 0.002041637357698527708, 0.003062456036547791995, 0.004083274715397057150, 0.006124912073095585725, 0.008166549430794116035 ),
 .UNSPECIFIED. ) ;
#2262=PLANE ( 'NONE',  #11284 ) ;
#2264=ORIENTED_EDGE ( 'NONE', *, *, #5545, .F. ) ;
#2267=ORIENTED_EDGE ( 'NONE', *, *, #2144, .T. ) ;
#2268=CARTESIAN_POINT ( 'NONE',  ( -24.99999999999998579, -99.17107372196666404, -0.8524342262974159423 ) ) ;
#2269=DIRECTION ( 'NONE',  ( -0.000000000000000000, -0.000000000000000000, -1.000000000000000000 ) ) ;
#2275=CARTESIAN_POINT ( 'NONE',  ( 2.449293598294706513E-15, -20.00000000000000000, -20.00000000000000000 ) ) ;
#2277=COLOUR_RGB ( '', 0.09019608, 0.27058824, 0.51372549) ;
#2284=VERTEX_POINT ( 'NONE', #9836 ) ;
#2285=ORIENTED_EDGE ( 'NONE', *, *, #5322, .T. ) ;
#2290=LINE ( 'NONE', #67, #9034 ) ;
#2298=DIRECTION ( 'NONE',  ( -1.224646799147353207E-16, 1.000000000000000000, -0.000000000000000000 ) ) ;
#2299=CARTESIAN_POINT ( 'NONE',  ( -34.99999999999999289, -135.0000000000000000, 0.000000000000000000 ) ) ;
#2304=EDGE_CURVE ( 'NONE', #11721, #8349, #2917, .T. ) ;
#2305=FACE_BOUND ( 'NONE', #914, .T. ) ;
#2314=EDGE_LOOP ( 'NONE', ( #9341, #1857, #7273, #600, #10836, #5625, #2107, #3019, #266, #847 ) ) ;
#2316=SURFACE_STYLE_USAGE ( .BOTH. , #9902 ) ;
#2317=VECTOR ( 'NONE', #10685, 1000.000000000000000 ) ;
#2320=CARTESIAN_POINT ( 'NONE',  ( 25.00000000000001776, -100.0000000000000000, 7.500000000000000000 ) ) ;
#2322=CARTESIAN_POINT ( 'NONE',  ( -24.99999999999998934, -100.0000000000000000, 5.046127144241784990 ) ) ;
#2324=CARTESIAN_POINT ( 'NONE',  ( -35.00000000000000000, -35.00000000000000000, 7.500000000000000000 ) ) ;
#2331=DIRECTION ( 'NONE',  ( -1.224646799147353207E-16, 1.000000000000000000, -0.000000000000000000 ) ) ;
#2342=SHAPE_REPRESENTATION ( 'Central Body Frame & Collar', ( #8193 ), #12229 ) ;
#2349=ORIENTED_EDGE ( 'NONE', *, *, #5228, .T. ) ;
#2352=ORIENTED_EDGE ( 'NONE', *, *, #7375, .F. ) ;
#2361=ORIENTED_EDGE ( 'NONE', *, *, #13309, .F. ) ;
#2362=AXIS2_PLACEMENT_3D ( 'NONE', #1763, #12652, #4139 ) ;
#2374=ORIENTED_EDGE ( 'NONE', *, *, #9852, .F. ) ;
#2378=FACE_OUTER_BOUND ( 'NONE', #12153, .T. ) ;
#2385=CARTESIAN_POINT ( 'NONE',  ( -35.00000000000012079, 91.25000000000045475, 4.000000000000000000 ) ) ;
#2392=VERTEX_POINT ( 'NONE', #3839 ) ;
#2396=ORIENTED_EDGE ( 'NONE', *, *, #11180, .F. ) ;
#2397=CARTESIAN_POINT ( 'NONE',  ( 0.000000000000000000, -100.0000000000000000, 0.000000000000000000 ) ) ;
#2408=EDGE_CURVE ( 'NONE', #4125, #5523, #8739, .T. ) ;
#2419=VECTOR ( 'NONE', #12974, 1000.000000000000000 ) ;
#2423=VERTEX_POINT ( 'NONE', #11748 ) ;
#2431=VERTEX_POINT ( 'NONE', #10562 ) ;
#2432=AXIS2_PLACEMENT_3D ( 'NONE', #13404, #2485, #12313 ) ;
#2437=ORIENTED_EDGE ( 'NONE', *, *, #2408, .F. ) ;
#2441=AXIS2_PLACEMENT_3D ( 'NONE', #10480, #2981, #9370 ) ;
#2448=ORIENTED_EDGE ( 'NONE', *, *, #3610, .F. ) ;
#2450=ORIENTED_EDGE ( 'NONE', *, *, #10971, .F. ) ;
#2451=ORIENTED_EDGE ( 'NONE', *, *, #3896, .T. ) ;
#2459=SURFACE_STYLE_FILL_AREA ( #1480 ) ;
#2461=CARTESIAN_POINT ( 'NONE',  ( -6.999999999999999112, -35.00000000000000000, 7.500000000000000000 ) ) ;
#2470=CARTESIAN_POINT ( 'NONE',  ( 35.00000000000000000, 4.286263797015736496E-15, 7.500000000000000000 ) ) ;
#2471=ADVANCED_FACE ( 'NONE', ( #7470 ), #7329, .F. ) ;
#2481=VERTEX_POINT ( 'NONE', #2927 ) ;
#2482=CARTESIAN_POINT ( 'NONE',  ( 0.000000000000000000, 20.00000000000000355, 0.000000000000000000 ) ) ;
#2485=DIRECTION ( 'NONE',  ( 0.000000000000000000, 1.000000000000000000, 0.000000000000000000 ) ) ;
#2492=TOROIDAL_SURFACE ( 'NONE', #4502, -34.24999999999974420, 69.24999999999975842 ) ;
#2493=CARTESIAN_POINT ( 'NONE',  ( -28.79177319725820894, -26.24642857144861807, -4.000000000000000000 ) ) ;
#2498=ORIENTED_EDGE ( 'NONE', *, *, #7796, .F. ) ;
#2505=LINE ( 'NONE', #10009, #10826 ) ;
#2514=SURFACE_SIDE_STYLE ('',( #2586 ) ) ;
#2518=ORIENTED_EDGE ( 'NONE', *, *, #13141, .T. ) ;
#2520=LINE ( 'NONE', #6797, #8685 ) ;
#2521=CARTESIAN_POINT ( 'NONE',  ( 20.00023673640404098, 26.72039747452867431, 1.279702169315402704 ) ) ;
#2526=ORIENTED_EDGE ( 'NONE', *, *, #4312, .F. ) ;
#2531=DIRECTION ( 'NONE',  ( 1.601283208593975514E-16, -1.000000000000000000, 0.000000000000000000 ) ) ;
#2542=FACE_OUTER_BOUND ( 'NONE', #11453, .T. ) ;
#2547=ORIENTED_EDGE ( 'NONE', *, *, #12196, .F. ) ;
#2549=ORIENTED_EDGE ( 'NONE', *, *, #8750, .T. ) ;
#2550=CIRCLE ( 'NONE', #10817, 14.99999999999999822 ) ;
#2556=VERTEX_POINT ( 'NONE', #5296 ) ;
#2557=ORIENTED_EDGE ( 'NONE', *, *, #2166, .T. ) ;
#2559=VERTEX_POINT ( 'NONE', #13889 ) ;
#2561=EDGE_CURVE ( 'NONE', #4208, #8094, #7388, .T. ) ;
#2565=PLANE ( 'NONE',  #7747 ) ;
#2569=VECTOR ( 'NONE', #975, 1000.000000000000000 ) ;
#2570=ORIENTED_EDGE ( 'NONE', *, *, #11064, .T. ) ;
#2572=VECTOR ( 'NONE', #12677, 1000.000000000000000 ) ;
#2577=VERTEX_POINT ( 'NONE', #11812 ) ;
#2586=SURFACE_STYLE_FILL_AREA ( #426 ) ;
#2595=CIRCLE ( 'NONE', #1464, 35.00000000000000000 ) ;
#2605=ORIENTED_EDGE ( 'NONE', *, *, #4535, .F. ) ;
#2609=ORIENTED_EDGE ( 'NONE', *, *, #3276, .T. ) ;
#2613=CARTESIAN_POINT ( 'NONE',  ( 1.922734475756564121E-15, 40.00000000000000000, -15.70031846811053455 ) ) ;
#2618=CARTESIAN_POINT ( 'NONE',  ( 35.00000000000000000, -4.286263797015736496E-15, -4.000000000000000000 ) ) ;
#2622=VECTOR ( 'NONE', #12188, 1000.000000000000000 ) ;
#2623=CARTESIAN_POINT ( 'NONE',  ( 35.00000000000001421, -34.99999999999999289, 7.500000000000000000 ) ) ;
#2624=ORIENTED_EDGE ( 'NONE', *, *, #628, .F. ) ;
#2640=AXIS2_PLACEMENT_3D ( 'NONE', #7358, #3152, #1066 ) ;
#2644=FACE_OUTER_BOUND ( 'NONE', #1184, .T. ) ;
#2652=ORIENTED_EDGE ( 'NONE', *, *, #4385, .F. ) ;
#2659=DIRECTION ( 'NONE',  ( 0.000000000000000000, 0.000000000000000000, 1.000000000000000000 ) ) ;
#2662=DIRECTION ( 'NONE',  ( 0.000000000000000000, 0.000000000000000000, 1.000000000000000000 ) ) ;
#2666=ORIENTED_EDGE ( 'NONE', *, *, #3262, .T. ) ;
#2670=AXIS2_PLACEMENT_3D ( 'NONE', #4014, #6327, #1073 ) ;
#2675=DIRECTION ( 'NONE',  ( 0.000000000000000000, 1.000000000000000000, 0.000000000000000000 ) ) ;
#2676=CARTESIAN_POINT ( 'NONE',  ( -23.09891356890233993, -97.97864346908494326, 7.500000000000000000 ) ) ;
#2680=CARTESIAN_POINT ( 'NONE',  ( -22.00000000000000000, -35.00000000000000000, 7.500000000000000000 ) ) ;
#2684=CYLINDRICAL_SURFACE ( 'NONE', #1034, 20.00000000000000000 ) ;
#2690=AXIS2_PLACEMENT_3D ( 'NONE', #11538, #9299, #3967 ) ;
#2695=DIRECTION ( 'NONE',  ( -0.000000000000000000, -0.000000000000000000, 1.000000000000000000 ) ) ;
#2700=AXIS2_PLACEMENT_3D ( 'NONE', #5599, #11709, #14 ) ;
#2717=CARTESIAN_POINT ( 'NONE',  ( 2.449293598294706513E-15, -20.00000000000000000, -20.00000000000000000 ) ) ;
#2718=DIRECTION ( 'NONE',  ( -1.224646799147353207E-16, 1.000000000000000000, -0.000000000000000000 ) ) ;
#2728=ORIENTED_EDGE ( 'NONE', *, *, #6920, .F. ) ;
#2738=DIRECTION ( 'NONE',  ( -1.224646799147353207E-16, 1.000000000000000000, -0.000000000000000000 ) ) ;
#2755=B_SPLINE_CURVE_WITH_KNOTS ( 'NONE', 3,
 ( #8424, #728, #10519, #9411, #9269, #9480, #13655, #10589, #3028, #9546, #13788, #1837, #10459, #7159, #13855, #4073 ),
 .UNSPECIFIED., .F., .F.,
 ( 4, 2, 2, 2, 2, 2, 2, 4 ),
 ( 0.000000000000000000, 0.003943481679486457968, 0.005915222519229687385, 0.007886963358972917670, 0.009858704198716147088, 0.01183044503845937477, 0.01380218587820260419, 0.01577392671794583534 ),
 .UNSPECIFIED. ) ;
#2765=LINE ( 'NONE', #4864, #12584 ) ;
#2768=PLANE ( 'NONE',  #8279 ) ;
#2781=EDGE_CURVE ( 'NONE', #3080, #3209, #11999, .T. ) ;
#2784=ORIENTED_EDGE ( 'NONE', *, *, #122, .T. ) ;
#2787=ORIENTED_EDGE ( 'NONE', *, *, #13704, .T. ) ;
#2790=CARTESIAN_POINT ( 'NONE',  ( -15.18222645069203303, -16.04698886238941924, -4.000000000000000000 ) ) ;
#2797=CARTESIAN_POINT ( 'NONE',  ( 32.50000000000000000, 4.286263797015736496E-15, 7.500000000000000000 ) ) ;
#2803=CYLINDRICAL_SURFACE ( 'NONE', #866, 31.93204061526060045 ) ;
#2827=VERTEX_POINT ( 'NONE', #10183 ) ;
#2832=EDGE_CURVE ( 'NONE', #8984, #13646, #5895, .T. ) ;
#2837=CARTESIAN_POINT ( 'NONE',  ( -13.79311422413708499, -21.62638421600851046, 7.500000000000000000 ) ) ;
#2838=DIRECTION ( 'NONE',  ( 0.000000000000000000, 1.000000000000000000, 0.000000000000000000 ) ) ;
#2841=CARTESIAN_POINT ( 'NONE',  ( 22.00000000000002132, -100.0000000000000000, 7.500000000000000000 ) ) ;
#2843=CARTESIAN_POINT ( 'NONE',  ( 35.00000000000000711, -25.00000000000000000, -7.500000000000000000 ) ) ;
#2847=ORIENTED_EDGE ( 'NONE', *, *, #11903, .T. ) ;
#2851=DIRECTION ( 'NONE',  ( 0.000000000000000000, 1.000000000000000000, 0.000000000000000000 ) ) ;
#2855=DIRECTION ( 'NONE',  ( 1.000000000000000000, 0.000000000000000000, 0.000000000000000000 ) ) ;
#2858=CIRCLE ( 'NONE', #2640, 23.64268088454700845 ) ;
#2862=ORIENTED_EDGE ( 'NONE', *, *, #5099, .F. ) ;
#2870=EDGE_CURVE ( 'NONE', #6184, #9446, #11513, .T. ) ;
#2872=CARTESIAN_POINT ( 'NONE',  ( -35.00000000000000000, -4.286263797015736496E-15, 4.000000000000000000 ) ) ;
#2879=CARTESIAN_POINT ( 'NONE',  ( 15.18222645069203303, -16.04698886238941924, -4.000000000000000000 ) ) ;
#2880=AXIS2_PLACEMENT_3D ( 'NONE', #777, #7419, #4977 ) ;
#2889=CARTESIAN_POINT ( 'NONE',  ( -35.00000000000000000, -35.00000000000000000, -7.500000000000000000 ) ) ;
#2891=PLANE ( 'NONE',  #9545 ) ;
#2894=ORIENTED_EDGE ( 'NONE', *, *, #8190, .F. ) ;
#2901=LINE ( 'NONE', #806, #4356 ) ;
#2903=CIRCLE ( 'NONE', #4912, 31.93204061526059334 ) ;
#2908=ADVANCED_FACE ( 'NONE', ( #4921 ), #12649, .F. ) ;
#2915=CIRCLE ( 'NONE', #681, 1.999999999999998224 ) ;
#2917=CIRCLE ( 'NONE', #8503, 15.70031846811053455 ) ;
#2922=CARTESIAN_POINT ( 'NONE',  ( 35.00000000000000711, -25.00000000000000000, -4.000000000000000000 ) ) ;
#2927=CARTESIAN_POINT ( 'NONE',  ( 25.00000000000001776, -99.15310334213020838, 3.061571689641656246E-15 ) ) ;
#2929=EDGE_CURVE ( 'NONE', #5523, #13483, #421, .T. ) ;
#2937=EDGE_LOOP ( 'NONE', ( #11427, #7187, #12929, #652, #2231 ) ) ;
#2938=VECTOR ( 'NONE', #9092, 1000.000000000000000 ) ;
#2953=VERTEX_POINT ( 'NONE', #4091 ) ;
#2970=ORIENTED_EDGE ( 'NONE', *, *, #7135, .T. ) ;
#2976=DIRECTION ( 'NONE',  ( -1.000000000000000000, 0.000000000000000000, 0.000000000000000000 ) ) ;
#2977=DIRECTION ( 'NONE',  ( 1.000000000000000000, 0.000000000000000000, 0.000000000000000000 ) ) ;
#2979=ORIENTED_EDGE ( 'NONE', *, *, #3269, .F. ) ;
#2981=DIRECTION ( 'NONE',  ( 0.000000000000000000, 0.000000000000000000, 1.000000000000000000 ) ) ;
#2985=EDGE_CURVE ( 'NONE', #3080, #2423, #12601, .T. ) ;
#2989=CARTESIAN_POINT ( 'NONE',  ( 14.10210168181666468, -21.78333407367942698, -6.931746760319976275 ) ) ;
#2996=VECTOR ( 'NONE', #4665, 1000.000000000000000 ) ;
#3003=CARTESIAN_POINT ( 'NONE',  ( -35.00000000000012079, 91.25000000000045475, 7.500000000000000000 ) ) ;
#3004=CARTESIAN_POINT ( 'NONE',  ( -60.00000000000001421, -4.286263797015736496E-15, -4.000000000000000000 ) ) ;
#3019=ORIENTED_EDGE ( 'NONE', *, *, #9530, .F. ) ;
#3025=EDGE_CURVE ( 'NONE', #4480, #6588, #54, .T. ) ;
#3028=CARTESIAN_POINT ( 'NONE',  ( -15.66041902283167175, -22.75225252538439236, 1.300500990791220168 ) ) ;
#3039=CIRCLE ( 'NONE', #4839, 2.500000000000002220 ) ;
#3040=DIRECTION ( 'NONE',  ( -0.000000000000000000, -0.000000000000000000, -1.000000000000000000 ) ) ;
#3045=CIRCLE ( 'NONE', #9315, 2.500000000000002220 ) ;
#3051=CARTESIAN_POINT ( 'NONE',  ( -35.00000000000000000, -4.286263797015736496E-15, -4.000000000000000000 ) ) ;
#3052=EDGE_LOOP ( 'NONE', ( #661, #11638, #2374, #7252, #7405, #6128, #12374, #9806, #2970, #716, #2728, #8460, #6000 ) ) ;
#3053=DIRECTION ( 'NONE',  ( 0.000000000000000000, 0.000000000000000000, 1.000000000000000000 ) ) ;
#3056=MANIFOLD_SOLID_BREP ( 'Fillet1', #2005 ) ;
#3058=DIRECTION ( 'NONE',  ( 0.000000000000000000, 1.000000000000000000, 0.000000000000000000 ) ) ;
#3066=ORIENTED_EDGE ( 'NONE', *, *, #3373, .T. ) ;
#3067=ORIENTED_EDGE ( 'NONE', *, *, #301, .T. ) ;
#3078=ORIENTED_EDGE ( 'NONE', *, *, #4460, .T. ) ;
#3080=VERTEX_POINT ( 'NONE', #3743 ) ;
#3092=CARTESIAN_POINT ( 'NONE',  ( 35.00000000000000000, 4.286263797015736496E-15, -4.000000000000000000 ) ) ;
#3095=ORIENTED_EDGE ( 'NONE', *, *, #540, .T. ) ;
#3097=EDGE_CURVE ( 'NONE', #2556, #9444, #12984, .T. ) ;
#3098=CIRCLE ( 'NONE', #199, 25.00000000000000355 ) ;
#3103=DIRECTION ( 'NONE',  ( -0.000000000000000000, 1.000000000000000000, -0.000000000000000000 ) ) ;
#3111=FACE_BOUND ( 'NONE', #12341, .T. ) ;
#3120=CARTESIAN_POINT ( 'NONE',  ( 35.00000000000009237, 91.25000000000046896, 7.500000000000000000 ) ) ;
#3127=VERTEX_POINT ( 'NONE', #6448 ) ;
#3134=CARTESIAN_POINT ( 'NONE',  ( 35.00000000000000000, 4.286263797015736496E-15, 7.500000000000000000 ) ) ;
#3140=AXIS2_PLACEMENT_3D ( 'NONE', #9537, #6699, #12766 ) ;
#3147=APPLICATION_CONTEXT ( 'automotive_design' ) ;
#3149=DIRECTION ( 'NONE',  ( 1.000000000000000000, 1.224646799147353207E-16, 0.000000000000000000 ) ) ;
#3151=CARTESIAN_POINT ( 'NONE',  ( -24.99999999999999289, -99.52837026979777590, 3.391106264173251450 ) ) ;
#3152=DIRECTION ( 'NONE',  ( -1.224646799147353207E-16, 1.000000000000000000, -0.000000000000000000 ) ) ;
#3153=CIRCLE ( 'NONE', #1810, 2.500000000000002220 ) ;
#3155=CARTESIAN_POINT ( 'NONE',  ( 25.00000000000001776, -100.0000000000000000, -7.500000000000000000 ) ) ;
#3164=ORIENTED_EDGE ( 'NONE', *, *, #3334, .F. ) ;
#3176=VERTEX_POINT ( 'NONE', #7763 ) ;
#3191=EDGE_CURVE ( 'NONE', #1947, #8894, #12921, .T. ) ;
#3202=CARTESIAN_POINT ( 'NONE',  ( 0.000000000000000000, -20.00000000000000000, 20.00000000000000000 ) ) ;
#3209=VERTEX_POINT ( 'NONE', #11907 ) ;
#3214=VERTEX_POINT ( 'NONE', #1258 ) ;
#3218=CARTESIAN_POINT ( 'NONE',  ( -35.00000000000000000, 25.00000000000000000, 4.000000000000000000 ) ) ;
#3226=CIRCLE ( 'NONE', #13113, 23.64268088454700845 ) ;
#3241=EDGE_CURVE ( 'NONE', #2953, #8273, #4688, .T. ) ;
#3243=CARTESIAN_POINT ( 'NONE',  ( -24.99999999999998934, -100.0000000000000000, -7.500000000000000000 ) ) ;
#3262=EDGE_CURVE ( 'NONE', #13056, #12412, #33, .T. ) ;
#3263=FACE_BOUND ( 'NONE', #13106, .T. ) ;
#3266=ADVANCED_FACE ( 'NONE', ( #12348 ), #3847, .F. ) ;
#3269=EDGE_CURVE ( 'NONE', #6682, #4795, #12795, .T. ) ;
#3273=DIRECTION ( 'NONE',  ( 0.000000000000000000, 0.000000000000000000, 1.000000000000000000 ) ) ;
#3276=EDGE_CURVE ( 'NONE', #1407, #13124, #7621, .T. ) ;
#3280=ORIENTED_EDGE ( 'NONE', *, *, #11093, .T. ) ;
#3281=EDGE_CURVE ( 'NONE', #3625, #3737, #1150, .T. ) ;
#3305=AXIS2_PLACEMENT_3D ( 'NONE', #4124, #8272, #2023 ) ;
#3306=ORIENTED_EDGE ( 'NONE', *, *, #8190, .T. ) ;
#3307=CIRCLE ( 'NONE', #2190, 22.00000000000000355 ) ;
#3308=DIRECTION ( 'NONE',  ( -1.000000000000000000, 0.000000000000000000, 0.000000000000000000 ) ) ;
#3309=DIRECTION ( 'NONE',  ( -0.000000000000000000, -0.000000000000000000, 1.000000000000000000 ) ) ;
#3311=DIRECTION ( 'NONE',  ( 0.000000000000000000, 0.000000000000000000, 1.000000000000000000 ) ) ;
#3312=FACE_OUTER_BOUND ( 'NONE', #6822, .T. ) ;
#3334=EDGE_CURVE ( 'NONE', #2559, #3663, #6972, .T. ) ;
#3337=AXIS2_PLACEMENT_3D ( 'NONE', #11385, #12246, #9227 ) ;
#3338=CARTESIAN_POINT ( 'NONE',  ( 25.00000000000002132, -99.17107372196666404, 0.8524342262973642059 ) ) ;
#3352=CARTESIAN_POINT ( 'NONE',  ( 35.00000000000000000, 4.286263797015736496E-15, -7.500000000000000000 ) ) ;
#3356=AXIS2_PLACEMENT_3D ( 'NONE', #7845, #4691, #3483 ) ;
#3366=ORIENTED_EDGE ( 'NONE', *, *, #6659, .F. ) ;
#3373=EDGE_CURVE ( 'NONE', #3769, #12961, #927, .T. ) ;
#3389=AXIS2_PLACEMENT_3D ( 'NONE', #10518, #9204, #8149 ) ;
#3397=ORIENTED_EDGE ( 'NONE', *, *, #543, .F. ) ;
#3398=CARTESIAN_POINT ( 'NONE',  ( -35.00000000000000000, -4.286263797015736496E-15, 4.000000000000000000 ) ) ;
#3399=ORIENTED_EDGE ( 'NONE', *, *, #12828, .F. ) ;
#3401=EDGE_LOOP ( 'NONE', ( #8208, #7217, #74, #1560 ) ) ;
#3403=DIRECTION ( 'NONE',  ( -0.000000000000000000, -1.000000000000000000, -0.000000000000000000 ) ) ;
#3411=AXIS2_PLACEMENT_3D ( 'NONE', #10087, #6785, #11137 ) ;
#3415=ORIENTED_EDGE ( 'NONE', *, *, #2985, .F. ) ;
#3432=DIRECTION ( 'NONE',  ( -0.000000000000000000, -0.000000000000000000, -1.000000000000000000 ) ) ;
#3433=VERTEX_POINT ( 'NONE', #11760 ) ;
#3441=AXIS2_PLACEMENT_3D ( 'NONE', #12258, #6914, #3834 ) ;
#3444=DIRECTION ( 'NONE',  ( 0.000000000000000000, 1.000000000000000000, 0.000000000000000000 ) ) ;
#3447=FACE_OUTER_BOUND ( 'NONE', #1254, .T. ) ;
#3453=DIRECTION ( 'NONE',  ( -1.000000000000000000, 0.000000000000000000, 0.000000000000000000 ) ) ;
#3464=VECTOR ( 'NONE', #249, 1000.000000000000000 ) ;
#3470=AXIS2_PLACEMENT_3D ( 'NONE', #12013, #7589, #9705 ) ;
#3472=CARTESIAN_POINT ( 'NONE',  ( 22.00000000000002132, -97.00000000000000000, 7.500000000000000000 ) ) ;
#3476=ORIENTED_EDGE ( 'NONE', *, *, #7609, .T. ) ;
#3478=ORIENTED_EDGE ( 'NONE', *, *, #4916, .T. ) ;
#3479=ORIENTED_EDGE ( 'NONE', *, *, #4535, .T. ) ;
#3483=DIRECTION ( 'NONE',  ( 0.000000000000000000, 0.000000000000000000, 1.000000000000000000 ) ) ;
#3488=VERTEX_POINT ( 'NONE', #327 ) ;
#3490=VERTEX_POINT ( 'NONE', #7804 ) ;
#3504=CARTESIAN_POINT ( 'NONE',  ( -15.18222645069203303, 20.00000000000000000, -4.000000000000000000 ) ) ;
#3515=CARTESIAN_POINT ( 'NONE',  ( -24.99999999999999289, -99.72710464630432625, -4.238242954203594870 ) ) ;
#3516=CARTESIAN_POINT ( 'NONE',  ( -30.72062512117240018, 25.13835616439069653, -4.000000000000000000 ) ) ;
#3517=EDGE_LOOP ( 'NONE', ( #13594, #12178, #4345, #11699 ) ) ;
#3527=CARTESIAN_POINT ( 'NONE',  ( -13.79311422413708499, -20.00000000000000355, 7.500000000000000000 ) ) ;
#3536=DIRECTION ( 'NONE',  ( -0.000000000000000000, -0.000000000000000000, -1.000000000000000000 ) ) ;
#3541=DIRECTION ( 'NONE',  ( 0.000000000000000000, 0.000000000000000000, 1.000000000000000000 ) ) ;
#3548=EDGE_CURVE ( 'NONE', #7192, #3769, #11237, .T. ) ;
#3549=PRESENTATION_STYLE_ASSIGNMENT (( #12121 ) ) ;
#3554=ORIENTED_EDGE ( 'NONE', *, *, #6621, .T. ) ;
#3555=DIRECTION ( 'NONE',  ( 0.000000000000000000, 0.000000000000000000, 1.000000000000000000 ) ) ;
#3559=DIRECTION ( 'NONE',  ( -0.000000000000000000, -0.000000000000000000, -1.000000000000000000 ) ) ;
#3570=ORIENTED_EDGE ( 'NONE', *, *, #9107, .F. ) ;
#3574=AXIS2_PLACEMENT_3D ( 'NONE', #6034, #11423, #4121 ) ;
#3581=DIRECTION ( 'NONE',  ( -0.000000000000000000, -0.000000000000000000, -1.000000000000000000 ) ) ;
#3588=ADVANCED_FACE ( 'NONE', ( #12314 ), #2492, .T. ) ;
#3610=EDGE_CURVE ( 'NONE', #10241, #12162, #1651, .T. ) ;
#3614=EDGE_CURVE ( 'NONE', #2577, #2559, #3889, .T. ) ;
#3615=ORIENTED_EDGE ( 'NONE', *, *, #452, .F. ) ;
#3622=CARTESIAN_POINT ( 'NONE',  ( -35.00000000000000000, -4.286263797015736496E-15, -7.500000000000000000 ) ) ;
#3625=VERTEX_POINT ( 'NONE', #10344 ) ;
#3626=VECTOR ( 'NONE', #9741, 1000.000000000000000 ) ;
#3632=DIRECTION ( 'NONE',  ( 0.000000000000000000, 1.000000000000000000, 0.000000000000000000 ) ) ;
#3642=VECTOR ( 'NONE', #6161, 1000.000000000000000 ) ;
#3651=AXIS2_PLACEMENT_3D ( 'NONE', #9676, #7636, #11845 ) ;
#3658=DIRECTION ( 'NONE',  ( -1.224646799147353207E-16, 1.000000000000000000, -0.000000000000000000 ) ) ;
#3663=VERTEX_POINT ( 'NONE', #11260 ) ;
#3679=CARTESIAN_POINT ( 'NONE',  ( -28.79177319725820894, -26.24642857144861807, 4.000000000000000000 ) ) ;
#3706=EDGE_LOOP ( 'NONE', ( #12113, #13753, #4595, #7319 ) ) ;
#3711=DIRECTION ( 'NONE',  ( 1.000000000000000000, 0.000000000000000000, 0.000000000000000000 ) ) ;
#3716=AXIS2_PLACEMENT_3D ( 'NONE', #5194, #8286, #12583 ) ;
#3724=CYLINDRICAL_SURFACE ( 'NONE', #2216, 2.500000000000002220 ) ;
#3732=DIRECTION ( 'NONE',  ( -1.000000000000000000, 0.000000000000000000, 0.000000000000000000 ) ) ;
#3735=CARTESIAN_POINT ( 'NONE',  ( 15.34998809918498353, -16.25417180422370933, -3.363251165709652213 ) ) ;
#3737=VERTEX_POINT ( 'NONE', #7445 ) ;
#3741=VERTEX_POINT ( 'NONE', #871 ) ;
#3743=CARTESIAN_POINT ( 'NONE',  ( -60.00000000000001421, -4.286263797015736496E-15, 7.500000000000000000 ) ) ;
#3749=DIRECTION ( 'NONE',  ( -0.000000000000000000, -0.000000000000000000, -1.000000000000000000 ) ) ;
#3756=FACE_OUTER_BOUND ( 'NONE', #12279, .T. ) ;
#3769=VERTEX_POINT ( 'NONE', #7244 ) ;
#3771=ORIENTED_EDGE ( 'NONE', *, *, #8007, .F. ) ;
#3777=EDGE_LOOP ( 'NONE', ( #12951, #8664, #12764, #13721 ) ) ;
#3779=DIRECTION ( 'NONE',  ( -1.224646799147353207E-16, 1.000000000000000000, -0.000000000000000000 ) ) ;
#3784=DIRECTION ( 'NONE',  ( 0.000000000000000000, -0.000000000000000000, 1.000000000000000000 ) ) ;
#3811=CIRCLE ( 'NONE', #11644, 15.70031846811053455 ) ;
#3815=CARTESIAN_POINT ( 'NONE',  ( 34.24999999999975842, -135.0000000000000000, 0.000000000000000000 ) ) ;
#3822=DIRECTION ( 'NONE',  ( 0.000000000000000000, 0.000000000000000000, 1.000000000000000000 ) ) ;
#3828=AXIS2_PLACEMENT_3D ( 'NONE', #7881, #2269, #13168 ) ;
#3829=ORIENTED_EDGE ( 'NONE', *, *, #5734, .F. ) ;
#3834=DIRECTION ( 'NONE',  ( 0.000000000000000000, 0.000000000000000000, 1.000000000000000000 ) ) ;
#3835=AXIS2_PLACEMENT_3D ( 'NONE', #104, #6604, #11866 ) ;
#3839=CARTESIAN_POINT ( 'NONE',  ( 34.99999999999999289, 25.00000000000002132, -4.000000000000000000 ) ) ;
#3845=EDGE_LOOP ( 'NONE', ( #5982, #12717, #3479, #5302 ) ) ;
#3847=PLANE ( 'NONE',  #6740 ) ;
#3850=LINE ( 'NONE', #8457, #7980 ) ;
#3854=EDGE_CURVE ( 'NONE', #8546, #6099, #12590, .T. ) ;
#3856=ORIENTED_EDGE ( 'NONE', *, *, #11155, .F. ) ;
#3857=ORIENTED_EDGE ( 'NONE', *, *, #6340, .F. ) ;
#3861=DIRECTION ( 'NONE',  ( 0.000000000000000000, 0.000000000000000000, -1.000000000000000000 ) ) ;
#3873=DIRECTION ( 'NONE',  ( -0.000000000000000000, -0.000000000000000000, -1.000000000000000000 ) ) ;
#3878=ORIENTED_EDGE ( 'NONE', *, *, #10140, .T. ) ;
#3889=LINE ( 'NONE', #4873, #12124 ) ;
#3893=CIRCLE ( 'NONE', #1420, 31.93204061526059334 ) ;
#3896=EDGE_CURVE ( 'NONE', #7690, #10314, #1760, .T. ) ;
#3916=B_SPLINE_CURVE_WITH_KNOTS ( 'NONE', 3,
 ( #1684, #6724, #12133, #581, #5969, #364, #10237, #2521, #4622, #10170, #4844, #11150, #8903, #4904 ),
 .UNSPECIFIED., .F., .F.,
 ( 4, 2, 2, 2, 2, 2, 4 ),
 ( 0.000000000000000000, 0.003826572935444120475, 0.005739859403166179194, 0.007653145870888239215, 0.01147971880633235665, 0.01339300527405441407, 0.01530629174177647149 ),
 .UNSPECIFIED. ) ;
#3917=ORIENTED_EDGE ( 'NONE', *, *, #3241, .T. ) ;
#3925=CARTESIAN_POINT ( 'NONE',  ( 0.000000000000000000, -20.00000000000000355, 0.000000000000000000 ) ) ;
#3927=ORIENTED_EDGE ( 'NONE', *, *, #10232, .T. ) ;
#3938=FACE_OUTER_BOUND ( 'NONE', #11047, .T. ) ;
#3939=PRODUCT_DEFINITION ( 'UNKNOWN', '', #9095, #10227 ) ;
#3942=FACE_OUTER_BOUND ( 'NONE', #2937, .T. ) ;
#3944=DIRECTION ( 'NONE',  ( 1.000000000000000000, 0.000000000000000000, 0.000000000000000000 ) ) ;
#3950=ADVANCED_FACE ( 'NONE', ( #13084 ), #12148, .F. ) ;
#3956=FACE_OUTER_BOUND ( 'NONE', #9915, .T. ) ;
#3963=CARTESIAN_POINT ( 'NONE',  ( -19.87806660956081473, 26.74843260078020890, -2.549167750534977017 ) ) ;
#3964=DIRECTION ( 'NONE',  ( 0.000000000000000000, 0.000000000000000000, 1.000000000000000000 ) ) ;
#3966=ORIENTED_EDGE ( 'NONE', *, *, #11903, .F. ) ;
#3967=DIRECTION ( 'NONE',  ( 1.601283208593975514E-16, -1.000000000000000000, 0.000000000000000000 ) ) ;
#3980=ORIENTED_EDGE ( 'NONE', *, *, #2062, .F. ) ;
#3992=ORIENTED_EDGE ( 'NONE', *, *, #3854, .T. ) ;
#3997=ORIENTED_EDGE ( 'NONE', *, *, #4608, .T. ) ;
#4007=VERTEX_POINT ( 'NONE', #2613 ) ;
#4012=CIRCLE ( 'NONE', #2432, 20.00000000000000000 ) ;
#4014=CARTESIAN_POINT ( 'NONE',  ( -35.00000000000000000, -4.286263797015736496E-15, 7.500000000000000000 ) ) ;
#4021=CIRCLE ( 'NONE', #2441, 25.50000000002550138 ) ;
#4031=ADVANCED_FACE ( 'NONE', ( #3938, #5763 ), #10117, .T. ) ;
#4038=DIRECTION ( 'NONE',  ( -0.000000000000000000, -0.000000000000000000, -1.000000000000000000 ) ) ;
#4048=ADVANCED_FACE ( 'NONE', ( #6951 ), #6887, .F. ) ;
#4049=ORIENTED_EDGE ( 'NONE', *, *, #628, .T. ) ;
#4062=ORIENTED_EDGE ( 'NONE', *, *, #2094, .F. ) ;
#4064=ORIENTED_EDGE ( 'NONE', *, *, #2408, .T. ) ;
#4069=VERTEX_POINT ( 'NONE', #4788 ) ;
#4073=CARTESIAN_POINT ( 'NONE',  ( -13.79311422413708499, -21.62638421600851046, 7.500000000000000000 ) ) ;
#4074=CARTESIAN_POINT ( 'NONE',  ( -60.00000000000001421, -4.286263797015736496E-15, -7.500000000000000000 ) ) ;
#4089=DIRECTION ( 'NONE',  ( -0.000000000000000000, -0.000000000000000000, -1.000000000000000000 ) ) ;
#4090=DIRECTION ( 'NONE',  ( -0.000000000000000000, -0.000000000000000000, 1.000000000000000000 ) ) ;
#4091=CARTESIAN_POINT ( 'NONE',  ( 24.37649275748779232, -100.0000000000000000, 7.500000000000000000 ) ) ;
#4098=VERTEX_POINT ( 'NONE', #8215 ) ;
#4104=CARTESIAN_POINT ( 'NONE',  ( 15.36839996672161668, -22.54980054760554964, 3.276782387371332650 ) ) ;
#4112=ORIENTED_EDGE ( 'NONE', *, *, #11471, .F. ) ;
#4113=AXIS2_PLACEMENT_3D ( 'NONE', #6072, #4090, #6214 ) ;
#4114=EDGE_CURVE ( 'NONE', #2431, #6056, #13210, .T. ) ;
#4115=EDGE_LOOP ( 'NONE', ( #3570, #162, #12231, #836, #10584, #2862, #659, #6283 ) ) ;
#4121=DIRECTION ( 'NONE',  ( -1.000000000000000000, -2.081668171172168119E-15, 0.000000000000000000 ) ) ;
#4124=CARTESIAN_POINT ( 'NONE',  ( -35.00000000000000000, -4.286263797015736496E-15, -7.500000000000000000 ) ) ;
#4125=VERTEX_POINT ( 'NONE', #11512 ) ;
#4127=AXIS2_PLACEMENT_3D ( 'NONE', #2461, #6741, #9973 ) ;
#4138=EDGE_CURVE ( 'NONE', #10241, #2392, #7571, .T. ) ;
#4139=DIRECTION ( 'NONE',  ( 1.000000000000000000, -1.734723475976808672E-15, 0.000000000000000000 ) ) ;
#4142=DIRECTION ( 'NONE',  ( 0.000000000000000000, 0.000000000000000000, 1.000000000000000000 ) ) ;
#4149=DIRECTION ( 'NONE',  ( -1.000000000000000000, 0.000000000000000000, 0.000000000000000000 ) ) ;
#4164=ORIENTED_EDGE ( 'NONE', *, *, #4460, .F. ) ;
#4169=DIRECTION ( 'NONE',  ( 0.000000000000000000, 0.000000000000000000, 1.000000000000000000 ) ) ;
#4181=LINE ( 'NONE', #5106, #1223 ) ;
#4183=CARTESIAN_POINT ( 'NONE',  ( -18.54049621773915746, 27.07720798311999388, 7.500000000000000000 ) ) ;
#4195=CARTESIAN_POINT ( 'NONE',  ( 1.616533774874506480E-14, -132.0000000000000000, 0.000000000000000000 ) ) ;
#4201=CARTESIAN_POINT ( 'NONE',  ( -24.99999999999998934, -100.0000000000000000, 5.046127144241784990 ) ) ;
#4208=VERTEX_POINT ( 'NONE', #12851 ) ;
#4210=EDGE_CURVE ( 'NONE', #7680, #3433, #9479, .T. ) ;
#4218=CARTESIAN_POINT ( 'NONE',  ( -35.00000000000000000, -4.286263797015736496E-15, -4.000000000000000000 ) ) ;
#4226=ORIENTED_EDGE ( 'NONE', *, *, #10140, .F. ) ;
#4235=VECTOR ( 'NONE', #9770, 1000.000000000000000 ) ;
#4246=CIRCLE ( 'NONE', #3356, 15.70031846811053455 ) ;
#4264=DIRECTION ( 'NONE',  ( -1.224646799147353207E-16, 1.000000000000000000, -0.000000000000000000 ) ) ;
#4312=EDGE_CURVE ( 'NONE', #12643, #13879, #10846, .T. ) ;
#4313=DIRECTION ( 'NONE',  ( -0.000000000000000000, -0.000000000000000000, -1.000000000000000000 ) ) ;
#4319=ORIENTED_EDGE ( 'NONE', *, *, #8468, .T. ) ;
#4323=CARTESIAN_POINT ( 'NONE',  ( -19.75162188639114902, 26.77857048203551926, 3.206191164072789590 ) ) ;
#4327=ORIENTED_EDGE ( 'NONE', *, *, #9869, .F. ) ;
#4337=ORIENTED_EDGE ( 'NONE', *, *, #4385, .T. ) ;
#4345=ORIENTED_EDGE ( 'NONE', *, *, #5693, .T. ) ;
#4347=FILL_AREA_STYLE_COLOUR ( '', #6392 ) ;
#4351=DIRECTION ( 'NONE',  ( -0.000000000000000000, -0.000000000000000000, -1.000000000000000000 ) ) ;
#4356=VECTOR ( 'NONE', #7172, 1000.000000000000000 ) ;
#4359=EDGE_CURVE ( 'NONE', #3176, #5520, #3307, .T. ) ;
#4373=DIRECTION ( 'NONE',  ( -1.000000000000000000, 0.000000000000000000, 0.000000000000000000 ) ) ;
#4377=CYLINDRICAL_SURFACE ( 'NONE', #10445, 2.500000000000002220 ) ;
#4380=DIRECTION ( 'NONE',  ( -0.000000000000000000, 0.000000000000000000, -1.000000000000000000 ) ) ;
#4385=EDGE_CURVE ( 'NONE', #9931, #3127, #10915, .T. ) ;
#4389=CARTESIAN_POINT ( 'NONE',  ( 25.00000000000001776, -99.24349759607916610, 1.707585965103451509 ) ) ;
#4398=LINE ( 'NONE', #7627, #13710 ) ;
#4408=ORIENTED_EDGE ( 'NONE', *, *, #269, .T. ) ;
#4411=ORIENTED_EDGE ( 'NONE', *, *, #10582, .T. ) ;
#4414=DIRECTION ( 'NONE',  ( -1.000000000000000000, 0.000000000000000000, 0.000000000000000000 ) ) ;
#4417=CARTESIAN_POINT ( 'NONE',  ( -24.99999999999998934, -100.0000000000000000, -7.500000000000000000 ) ) ;
#4420=CYLINDRICAL_SURFACE ( 'NONE', #3835, 25.00000000000000355 ) ;
#4422=AXIS2_PLACEMENT_3D ( 'NONE', #3925, #12489, #5179 ) ;
#4433=CARTESIAN_POINT ( 'NONE',  ( 35.00000000000000000, 4.286263797015736496E-15, -7.500000000000000000 ) ) ;
#4443=PLANE ( 'NONE',  #6472 ) ;
#4445=DIRECTION ( 'NONE',  ( 0.000000000000000000, 0.000000000000000000, 1.000000000000000000 ) ) ;
#4446=AXIS2_PLACEMENT_3D ( 'NONE', #9899, #3432, #11990 ) ;
#4460=EDGE_CURVE ( 'NONE', #5520, #3176, #6018, .T. ) ;
#4467=VERTEX_POINT ( 'NONE', #709 ) ;
#4471=ADVANCED_FACE ( 'NONE', ( #10236 ), #2803, .F. ) ;
#4480=VERTEX_POINT ( 'NONE', #640 ) ;
#4487=AXIS2_PLACEMENT_3D ( 'NONE', #2470, #11017, #1156 ) ;
#4491=( NAMED_UNIT ( * ) SI_UNIT ( $, .STERADIAN. ) SOLID_ANGLE_UNIT ( ) );
#4495=AXIS2_PLACEMENT_3D ( 'NONE', #2397, #11803, #5419 ) ;
#4499=LINE ( 'NONE', #5622, #12354 ) ;
#4502=AXIS2_PLACEMENT_3D ( 'NONE', #1578, #1778, #5010 ) ;
#4505=DIRECTION ( 'NONE',  ( 0.000000000000000000, 1.000000000000000000, 0.000000000000000000 ) ) ;
#4507=CARTESIAN_POINT ( 'NONE',  ( 0.000000000000000000, 40.00000000000000000, 15.70031846811053455 ) ) ;
#4523=CARTESIAN_POINT ( 'NONE',  ( -6.999999999999999112, -35.00000000000000000, -7.500000000000000000 ) ) ;
#4525=CARTESIAN_POINT ( 'NONE',  ( 25.00000000000002487, -99.29838587104471515, 2.138129719433864206 ) ) ;
#4527=DIRECTION ( 'NONE',  ( -0.000000000000000000, -0.000000000000000000, 1.000000000000000000 ) ) ;
#4532=AXIS2_PLACEMENT_3D ( 'NONE', #2042, #7432, #8172 ) ;
#4535=EDGE_CURVE ( 'NONE', #4795, #4098, #2520, .T. ) ;
#4537=CARTESIAN_POINT ( 'NONE',  ( -25.00000000000000000, -35.00000000000000000, 7.500000000000000000 ) ) ;
#4549=ORIENTED_EDGE ( 'NONE', *, *, #6765, .T. ) ;
#4556=ORIENTED_EDGE ( 'NONE', *, *, #7807, .F. ) ;
#4563=CARTESIAN_POINT ( 'NONE',  ( 35.00000000000009237, 91.25000000000046896, 7.500000000000000000 ) ) ;
#4567=FACE_BOUND ( 'NONE', #6391, .T. ) ;
#4572=DIRECTION ( 'NONE',  ( 0.000000000000000000, 0.000000000000000000, 1.000000000000000000 ) ) ;
#4581=ADVANCED_FACE ( 'NONE', ( #13839 ), #11561, .T. ) ;
#4595=ORIENTED_EDGE ( 'NONE', *, *, #5545, .T. ) ;
#4607=FACE_OUTER_BOUND ( 'NONE', #3517, .T. ) ;
#4608=EDGE_CURVE ( 'NONE', #9044, #5648, #6240, .T. ) ;
#4609=UNCERTAINTY_MEASURE_WITH_UNIT (LENGTH_MEASURE( 1.000000000000000082E-05 ), #4684, 'distance_accuracy_value', 'NONE');
#4618=ORIENTED_EDGE ( 'NONE', *, *, #301, .F. ) ;
#4620=VECTOR ( 'NONE', #3273, 1000.000000000000000 ) ;
#4622=CARTESIAN_POINT ( 'NONE',  ( 19.87806660956081828, 26.74843260078022311, 2.549167750534976573 ) ) ;
#4625=EDGE_CURVE ( 'NONE', #13124, #6696, #841, .T. ) ;
#4627=ORIENTED_EDGE ( 'NONE', *, *, #11484, .F. ) ;
#4635=CARTESIAN_POINT ( 'NONE',  ( 22.00000000000002132, -97.00000000000000000, -7.500000000000000000 ) ) ;
#4649=EDGE_CURVE ( 'NONE', #6457, #2481, #919, .T. ) ;
#4651=DIRECTION ( 'NONE',  ( -0.000000000000000000, -0.000000000000000000, -1.000000000000000000 ) ) ;
#4665=DIRECTION ( 'NONE',  ( -5.337610695313252124E-17, 1.000000000000000000, 0.000000000000000000 ) ) ;
#4684=( LENGTH_UNIT ( ) NAMED_UNIT ( * ) SI_UNIT ( .MILLI., .METRE. ) );
#4686=EDGE_LOOP ( 'NONE', ( #5289, #2437 ) ) ;
#4688=LINE ( 'NONE', #9045, #8098 ) ;
#4690=DIRECTION ( 'NONE',  ( -1.000000000000000000, 0.000000000000000000, 0.000000000000000000 ) ) ;
#4691=DIRECTION ( 'NONE',  ( 0.000000000000000000, 1.000000000000000000, 0.000000000000000000 ) ) ;
#4695=ORIENTED_EDGE ( 'NONE', *, *, #8468, .F. ) ;
#4699=VECTOR ( 'NONE', #6735, 1000.000000000000000 ) ;
#4703=CARTESIAN_POINT ( 'NONE',  ( -22.42156014662057473, -97.00000000000000000, 7.500000000000000000 ) ) ;
#4710=DIRECTION ( 'NONE',  ( 1.000000000000000000, 0.000000000000000000, 0.000000000000000000 ) ) ;
#4725=AXIS2_PLACEMENT_3D ( 'NONE', #10208, #11389, #5013 ) ;
#4726=AXIS2_PLACEMENT_3D ( 'NONE', #4841, #7922, #1392 ) ;
#4727=EDGE_CURVE ( 'NONE', #13879, #3176, #5372, .T. ) ;
#4736=CARTESIAN_POINT ( 'NONE',  ( 35.00000000000000000, 4.286263797015736496E-15, 7.500000000000000000 ) ) ;
#4739=EDGE_CURVE ( 'NONE', #13646, #8612, #8741, .T. ) ;
#4742=CARTESIAN_POINT ( 'NONE',  ( 0.000000000000000000, -20.00000000000000355, 0.000000000000000000 ) ) ;
#4743=CARTESIAN_POINT ( 'NONE',  ( -18.78199004159287711, 27.01526789321293620, -6.903011289631056258 ) ) ;
#4744=CARTESIAN_POINT ( 'NONE',  ( 7.000000000000007994, -35.00000000000000000, 7.500000000000000000 ) ) ;
#4753=ORIENTED_EDGE ( 'NONE', *, *, #6685, .T. ) ;
#4755=AXIS2_PLACEMENT_3D ( 'NONE', #1017, #6791, #4766 ) ;
#4763=UNCERTAINTY_MEASURE_WITH_UNIT (LENGTH_MEASURE( 1.000000000000000082E-05 ), #7860, 'distance_accuracy_value', 'NONE');
#4765=ORIENTED_EDGE ( 'NONE', *, *, #5567, .T. ) ;
#4766=DIRECTION ( 'NONE',  ( -1.000000000000000000, 0.000000000000000000, 0.000000000000000000 ) ) ;
#4769=EDGE_LOOP ( 'NONE', ( #12214, #1769, #4226, #4894 ) ) ;
#4780=AXIS2_PLACEMENT_3D ( 'NONE', #8796, #8722, #2206 ) ;
#4781=ORIENTED_EDGE ( 'NONE', *, *, #4983, .T. ) ;
#4782=CARTESIAN_POINT ( 'NONE',  ( 0.000000000000000000, -20.00000000000000000, 20.00000000000000000 ) ) ;
#4784=EDGE_LOOP ( 'NONE', ( #8057, #4753, #12087, #6836, #3366 ) ) ;
#4788=CARTESIAN_POINT ( 'NONE',  ( 0.000000000000000000, -20.00000000000000355, 15.70031846811053455 ) ) ;
#4792=CARTESIAN_POINT ( 'NONE',  ( 15.70027825049740500, -16.66645554390144568, 0.3441452025673427118 ) ) ;
#4795=VERTEX_POINT ( 'NONE', #10159 ) ;
#4796=EDGE_CURVE ( 'NONE', #8273, #6184, #7828, .T. ) ;
#4805=ORIENTED_EDGE ( 'NONE', *, *, #7623, .F. ) ;
#4813=DIRECTION ( 'NONE',  ( 0.000000000000000000, 0.000000000000000000, 1.000000000000000000 ) ) ;
#4815=EDGE_CURVE ( 'NONE', #2827, #8984, #13633, .T. ) ;
#4818=VECTOR ( 'NONE', #6949, 1000.000000000000000 ) ;
#4836=ORIENTED_EDGE ( 'NONE', *, *, #2166, .F. ) ;
#4838=EDGE_CURVE ( 'NONE', #6056, #3127, #9035, .T. ) ;
#4839=AXIS2_PLACEMENT_3D ( 'NONE', #12430, #7094, #11302 ) ;
#4841=CARTESIAN_POINT ( 'NONE',  ( 35.00000000000001421, -34.99999999999999289, 4.000000000000000000 ) ) ;
#4844=CARTESIAN_POINT ( 'NONE',  ( 19.36040733361900124, 26.87219970003946656, 5.058700639371029872 ) ) ;
#4848=CIRCLE ( 'NONE', #12689, 2.500000000000002220 ) ;
#4851=EDGE_CURVE ( 'NONE', #2577, #7989, #13422, .T. ) ;
#4855=VERTEX_POINT ( 'NONE', #6858 ) ;
#4864=CARTESIAN_POINT ( 'NONE',  ( 22.00000000000002132, -97.00000000000000000, 7.500000000000000000 ) ) ;
#4870=CARTESIAN_POINT ( 'NONE',  ( 22.42156014662059249, -97.00000000000000000, -7.500000000000000000 ) ) ;
#4873=CARTESIAN_POINT ( 'NONE',  ( -18.54049621773915746, -20.00000000000000000, 7.500000000000000000 ) ) ;
#4874=FACE_OUTER_BOUND ( 'NONE', #12736, .T. ) ;
#4882=ORIENTED_EDGE ( 'NONE', *, *, #6789, .F. ) ;
#4885=CARTESIAN_POINT ( 'NONE',  ( -15.47908363509431595, -16.40738050097609602, -2.711248065311635091 ) ) ;
#4889=CARTESIAN_POINT ( 'NONE',  ( 27.38873514654796537, -24.33759740261775661, -4.000000000000000000 ) ) ;
#4894=ORIENTED_EDGE ( 'NONE', *, *, #4815, .F. ) ;
#4895=VECTOR ( 'NONE', #12371, 1000.000000000000000 ) ;
#4904=CARTESIAN_POINT ( 'NONE',  ( 18.54049621773915746, 27.07720798312000809, 7.500000000000000000 ) ) ;
#4912=AXIS2_PLACEMENT_3D ( 'NONE', #12791, #13799, #4149 ) ;
#4916=EDGE_CURVE ( 'NONE', #6758, #6312, #10361, .T. ) ;
#4921=FACE_OUTER_BOUND ( 'NONE', #13635, .T. ) ;
#4924=CARTESIAN_POINT ( 'NONE',  ( 25.00000000000001776, -100.0000000000000000, 7.500000000000000000 ) ) ;
#4925=AXIS2_PLACEMENT_3D ( 'NONE', #11461, #5011, #1921 ) ;
#4926=LINE ( 'NONE', #9136, #4895 ) ;
#4932=DIRECTION ( 'NONE',  ( 0.000000000000000000, 0.000000000000000000, 1.000000000000000000 ) ) ;
#4944=FACE_OUTER_BOUND ( 'NONE', #6413, .T. ) ;
#4949=AXIS2_PLACEMENT_3D ( 'NONE', #10473, #13676, #877 ) ;
#4953=ORIENTED_EDGE ( 'NONE', *, *, #12001, .F. ) ;
#4962=AXIS2_PLACEMENT_3D ( 'NONE', #12376, #9074, #12233 ) ;
#4965=DIRECTION ( 'NONE',  ( -0.000000000000000000, 1.000000000000000000, -0.000000000000000000 ) ) ;
#4977=DIRECTION ( 'NONE',  ( -1.000000000000000000, 0.000000000000000000, 0.000000000000000000 ) ) ;
#4983=EDGE_CURVE ( 'NONE', #8546, #1355, #1266, .T. ) ;
#4987=ORIENTED_EDGE ( 'NONE', *, *, #4114, .F. ) ;
#4994=AXIS2_PLACEMENT_3D ( 'NONE', #13114, #1113, #277 ) ;
#4996=AXIS2_PLACEMENT_3D ( 'NONE', #2140, #4313, #8594 ) ;
#5007=DIRECTION ( 'NONE',  ( -1.000000000000000000, 0.000000000000000000, 0.000000000000000000 ) ) ;
#5010=DIRECTION ( 'NONE',  ( -1.000000000000000000, -1.224646799147353207E-16, 0.000000000000000000 ) ) ;
#5011=DIRECTION ( 'NONE',  ( 0.000000000000000000, 0.000000000000000000, 1.000000000000000000 ) ) ;
#5013=DIRECTION ( 'NONE',  ( 0.000000000000000000, 0.000000000000000000, 1.000000000000000000 ) ) ;
#5016=VERTEX_POINT ( 'NONE', #8794 ) ;
#5017=PLANE ( 'NONE',  #2690 ) ;
#5025=CARTESIAN_POINT ( 'NONE',  ( -15.18222645069203303, -16.04698886238941924, 4.000000000000000000 ) ) ;
#5026=CARTESIAN_POINT ( 'NONE',  ( 15.65828099947304253, -22.75074427536019783, 1.322318745440853593 ) ) ;
#5039=AXIS2_PLACEMENT_3D ( 'NONE', #4736, #3749, #8032 ) ;
#5040=LINE ( 'NONE', #7863, #766 ) ;
#5042=CARTESIAN_POINT ( 'NONE',  ( 26.79177319725820539, -26.24642857144861807, -4.000000000000000000 ) ) ;
#5045=FACE_OUTER_BOUND ( 'NONE', #12481, .T. ) ;
#5049=ORIENTED_EDGE ( 'NONE', *, *, #3191, .T. ) ;
#5059=DIRECTION ( 'NONE',  ( -1.224646799147353207E-16, 1.000000000000000000, -0.000000000000000000 ) ) ;
#5068=DIRECTION ( 'NONE',  ( -1.224646799147353207E-16, 1.000000000000000000, -0.000000000000000000 ) ) ;
#5086=ADVANCED_FACE ( 'NONE', ( #9924, #8871 ), #2565, .F. ) ;
#5097=DIRECTION ( 'NONE',  ( 0.000000000000000000, 0.000000000000000000, 1.000000000000000000 ) ) ;
#5099=EDGE_CURVE ( 'NONE', #4069, #3488, #9557, .T. ) ;
#5106=CARTESIAN_POINT ( 'NONE',  ( -37.50000000000000711, -4.286263797015736496E-15, 7.500000000000000000 ) ) ;
#5124=CARTESIAN_POINT ( 'NONE',  ( 22.00000000000002132, -100.0000000000000000, 7.500000000000000000 ) ) ;
#5127=ORIENTED_EDGE ( 'NONE', *, *, #2832, .T. ) ;
#5149=LINE ( 'NONE', #3243, #5364 ) ;
#5153=ORIENTED_EDGE ( 'NONE', *, *, #2781, .T. ) ;
#5155=CARTESIAN_POINT ( 'NONE',  ( -27.38873514654796537, -24.33759740261776017, -4.000000000000000000 ) ) ;
#5161=CARTESIAN_POINT ( 'NONE',  ( 14.88155114952949276, -22.23162151614121029, 5.171026666816163520 ) ) ;
#5164=DIRECTION ( 'NONE',  ( -5.337610695313252124E-17, 1.000000000000000000, 0.000000000000000000 ) ) ;
#5171=CIRCLE ( 'NONE', #13014, 14.99999999999999822 ) ;
#5179=DIRECTION ( 'NONE',  ( 0.000000000000000000, 0.000000000000000000, 1.000000000000000000 ) ) ;
#5187=ORIENTED_EDGE ( 'NONE', *, *, #4851, .F. ) ;
#5194=CARTESIAN_POINT ( 'NONE',  ( 0.000000000000000000, -100.0000000000000000, 0.000000000000000000 ) ) ;
#5198=EDGE_LOOP ( 'NONE', ( #11587, #9300, #9779, #11473 ) ) ;
#5204=VECTOR ( 'NONE', #8792, 1000.000000000000000 ) ;
#5222=DIRECTION ( 'NONE',  ( -1.000000000000000000, 0.000000000000000000, 0.000000000000000000 ) ) ;
#5225=EDGE_CURVE ( 'NONE', #11226, #12718, #2169, .T. ) ;
#5228=EDGE_CURVE ( 'NONE', #9113, #2556, #2858, .T. ) ;
#5235=TOROIDAL_SURFACE ( 'NONE', #328, -34.24999999999974420, 66.24999999999978684 ) ;
#5242=CIRCLE ( 'NONE', #9507, 2.000000000000001776 ) ;
#5245=DIRECTION ( 'NONE',  ( 0.000000000000000000, 0.000000000000000000, 1.000000000000000000 ) ) ;
#5255=ORIENTED_EDGE ( 'NONE', *, *, #11471, .T. ) ;
#5258=LINE ( 'NONE', #10325, #12782 ) ;
#5268=ORIENTED_EDGE ( 'NONE', *, *, #2209, .T. ) ;
#5282=CARTESIAN_POINT ( 'NONE',  ( 25.00000000000001421, -99.15310334213019416, -0.8520627238942191095 ) ) ;
#5286=CARTESIAN_POINT ( 'NONE',  ( 0.000000000000000000, -20.00000000000000000, 0.000000000000000000 ) ) ;
#5289=ORIENTED_EDGE ( 'NONE', *, *, #9614, .F. ) ;
#5291=ORIENTED_EDGE ( 'NONE', *, *, #5466, .T. ) ;
#5296=CARTESIAN_POINT ( 'NONE',  ( -22.42156014662057473, -97.00000000000000000, -7.500000000000000000 ) ) ;
#5302=ORIENTED_EDGE ( 'NONE', *, *, #6430, .T. ) ;
#5306=EDGE_CURVE ( 'NONE', #7989, #4069, #9702, .T. ) ;
#5308=DIRECTION ( 'NONE',  ( 1.000000000000000000, 0.000000000000000000, 0.000000000000000000 ) ) ;
#5315=ORIENTED_EDGE ( 'NONE', *, *, #7900, .F. ) ;
#5322=EDGE_CURVE ( 'NONE', #12944, #9535, #12714, .T. ) ;
#5334=ORIENTED_EDGE ( 'NONE', *, *, #8399, .F. ) ;
#5336=AXIS2_PLACEMENT_3D ( 'NONE', #1761, #10250, #5909 ) ;
#5344=CARTESIAN_POINT ( 'NONE',  ( 35.00000000000000000, 4.286263797015736496E-15, 7.500000000000000000 ) ) ;
#5360=DIRECTION ( 'NONE',  ( -0.000000000000000000, -0.000000000000000000, -1.000000000000000000 ) ) ;
#5364=VECTOR ( 'NONE', #2191, 1000.000000000000000 ) ;
#5367=AXIS2_PLACEMENT_3D ( 'NONE', #6875, #13363, #3711 ) ;
#5372=LINE ( 'NONE', #3472, #4620 ) ;
#5374=CARTESIAN_POINT ( 'NONE',  ( 23.10070469010960537, -97.98123128958475547, 7.500000000000000000 ) ) ;
#5383=ORIENTED_EDGE ( 'NONE', *, *, #11920, .F. ) ;
#5391=B_SPLINE_CURVE_WITH_KNOTS ( 'NONE', 3,
 ( #4183, #5442, #9662, #4323, #8604, #9730, #332, #7811, #3963, #12392, #552, #7181, #4743, #1657 ),
 .UNSPECIFIED., .F., .F.,
 ( 4, 2, 2, 2, 2, 2, 4 ),
 ( 0.000000000000000000, 0.003826572935444120041, 0.005739859403166178327, 0.007653145870888238347, 0.01147971880633235318, 0.01339300527405441234, 0.01530629174177646976 ),
 .UNSPECIFIED. ) ;
#5399=ADVANCED_FACE ( 'NONE', ( #12987 ), #9745, .F. ) ;
#5407=CARTESIAN_POINT ( 'NONE',  ( 22.00000000000002132, -97.00000000000000000, 7.500000000000000000 ) ) ;
#5412=LINE ( 'NONE', #7719, #10544 ) ;
#5418=ORIENTED_EDGE ( 'NONE', *, *, #12510, .F. ) ;
#5419=DIRECTION ( 'NONE',  ( 0.000000000000000000, 0.000000000000000000, 1.000000000000000000 ) ) ;
#5423=CARTESIAN_POINT ( 'NONE',  ( -60.00000000000001421, 20.00000000000000000, 4.000000000000000000 ) ) ;
#5425=DIRECTION ( 'NONE',  ( 1.000000000000000000, 0.000000000000000000, 0.000000000000000000 ) ) ;
#5430=CIRCLE ( 'NONE', #13316, 25.00000000000000355 ) ;
#5435=CIRCLE ( 'NONE', #1867, 15.00000000000000000 ) ;
#5442=CARTESIAN_POINT ( 'NONE',  ( -19.02348910326480436, 26.95332645987220133, 6.306009631028898887 ) ) ;
#5466=EDGE_CURVE ( 'NONE', #4467, #3741, #10996, .T. ) ;
#5468=FACE_OUTER_BOUND ( 'NONE', #7722, .T. ) ;
#5473=PRESENTATION_STYLE_ASSIGNMENT (( #2316 ) ) ;
#5481=CARTESIAN_POINT ( 'NONE',  ( 35.00000000000000711, -25.00000000000000000, 4.000000000000000000 ) ) ;
#5492=ORIENTED_EDGE ( 'NONE', *, *, #3025, .T. ) ;
#5496=CARTESIAN_POINT ( 'NONE',  ( -13.79311422413708499, -100.0000000000000000, -7.500000000000000000 ) ) ;
#5515=DIRECTION ( 'NONE',  ( 1.000000000000000000, 0.000000000000000000, 0.000000000000000000 ) ) ;
#5517=FACE_BOUND ( 'NONE', #8418, .T. ) ;
#5520=VERTEX_POINT ( 'NONE', #2153 ) ;
#5522=DIRECTION ( 'NONE',  ( 1.601283208593975514E-16, -1.000000000000000000, 0.000000000000000000 ) ) ;
#5523=VERTEX_POINT ( 'NONE', #348 ) ;
#5529=DIRECTION ( 'NONE',  ( 1.000000000000000000, -0.000000000000000000, -0.000000000000000000 ) ) ;
#5536=CARTESIAN_POINT ( 'NONE',  ( 34.99999999999999289, 25.00000000000002132, -7.500000000000000000 ) ) ;
#5538=FACE_OUTER_BOUND ( 'NONE', #13307, .T. ) ;
#5539=DIRECTION ( 'NONE',  ( -1.000000000000000000, 0.000000000000000000, 0.000000000000000000 ) ) ;
#5545=EDGE_CURVE ( 'NONE', #11430, #8708, #2290, .T. ) ;
#5546=AXIS2_PLACEMENT_3D ( 'NONE', #2618, #9273, #11096 ) ;
#5560=DIRECTION ( 'NONE',  ( -0.000000000000000000, -0.000000000000000000, -1.000000000000000000 ) ) ;
#5567=EDGE_CURVE ( 'NONE', #10692, #2953, #12602, .T. ) ;
#5569=ORIENTED_EDGE ( 'NONE', *, *, #6532, .F. ) ;
#5580=DIRECTION ( 'NONE',  ( -0.000000000000000000, -0.000000000000000000, -1.000000000000000000 ) ) ;
#5582=CARTESIAN_POINT ( 'NONE',  ( 25.00000000000001421, -99.72710464630424099, 4.238242954203321311 ) ) ;
#5586=EDGE_LOOP ( 'NONE', ( #11772, #2609, #11900, #1390 ) ) ;
#5588=ADVANCED_FACE ( 'NONE', ( #4607 ), #9873, .T. ) ;
#5592=AXIS2_PLACEMENT_3D ( 'NONE', #12708, #8417, #7348 ) ;
#5599=CARTESIAN_POINT ( 'NONE',  ( -35.00000000000012079, 91.25000000000045475, 7.500000000000000000 ) ) ;
#5610=ADVANCED_FACE ( 'NONE', ( #7754 ), #8888, .F. ) ;
#5622=CARTESIAN_POINT ( 'NONE',  ( -27.38873514654796537, -24.33759740261775661, -4.000000000000000000 ) ) ;
#5624=ORIENTED_EDGE ( 'NONE', *, *, #11526, .T. ) ;
#5625=ORIENTED_EDGE ( 'NONE', *, *, #10382, .F. ) ;
#5626=AXIS2_PLACEMENT_3D ( 'NONE', #8034, #809, #12245 ) ;
#5627=LINE ( 'NONE', #9986, #472 ) ;
#5629=CARTESIAN_POINT ( 'NONE',  ( -24.99999999999998934, -99.24349759607916610, -1.707585965103561865 ) ) ;
#5630=DIRECTION ( 'NONE',  ( -1.000000000000000000, 0.000000000000000000, 0.000000000000000000 ) ) ;
#5631=ORIENTED_EDGE ( 'NONE', *, *, #6703, .F. ) ;
#5634=ORIENTED_EDGE ( 'NONE', *, *, #1897, .F. ) ;
#5646=ORIENTED_EDGE ( 'NONE', *, *, #7631, .F. ) ;
#5648=VERTEX_POINT ( 'NONE', #9800 ) ;
#5663=VERTEX_POINT ( 'NONE', #142 ) ;
#5669=LINE ( 'NONE', #8860, #13249 ) ;
#5679=CARTESIAN_POINT ( 'NONE',  ( -25.00000000000000000, -35.00000000000000000, 7.500000000000000000 ) ) ;
#5681=ORIENTED_EDGE ( 'NONE', *, *, #543, .T. ) ;
#5683=CIRCLE ( 'NONE', #13354, 66.25000000000044054 ) ;
#5686=VERTEX_POINT ( 'NONE', #1672 ) ;
#5693=EDGE_CURVE ( 'NONE', #11449, #1592, #5430, .T. ) ;
#5695=VECTOR ( 'NONE', #6366, 1000.000000000000000 ) ;
#5698=CIRCLE ( 'NONE', #7482, 2.500000000000002220 ) ;
#5701=VECTOR ( 'NONE', #11543, 1000.000000000000000 ) ;
#5712=B_SPLINE_CURVE_WITH_KNOTS ( 'NONE', 3,
 ( #1488, #7944, #12228, #10048, #10255, #6889, #4792, #9069, #11169, #12431, #3735, #8019 ),
 .UNSPECIFIED., .F., .F.,
 ( 4, 2, 2, 2, 2, 4 ),
 ( 0.000000000000000000, 0.002041637357698527708, 0.003062456036547791995, 0.004083274715397057150, 0.006124912073095585725, 0.008166549430794116035 ),
 .UNSPECIFIED. ) ;
#5724=VERTEX_POINT ( 'NONE', #9169 ) ;
#5734=EDGE_CURVE ( 'NONE', #3663, #7690, #10226, .T. ) ;
#5740=DIRECTION ( 'NONE',  ( 1.000000000000000000, 0.000000000000000000, 0.000000000000000000 ) ) ;
#5744=CYLINDRICAL_SURFACE ( 'NONE', #13615, 25.50000000002550138 ) ;
#5763=FACE_BOUND ( 'NONE', #934, .T. ) ;
#5766=B_SPLINE_CURVE_WITH_KNOTS ( 'NONE', 3,
 ( #7734, #10953, #9781, #325 ),
 .UNSPECIFIED., .F., .F.,
 ( 4, 4 ),
 ( 0.02301878569831470461, 0.02656428146801016396 ),
 .UNSPECIFIED. ) ;
#5769=ORIENTED_EDGE ( 'NONE', *, *, #8067, .F. ) ;
#5771=EDGE_CURVE ( 'NONE', #11226, #11483, #11928, .T. ) ;
#5777=CARTESIAN_POINT ( 'NONE',  ( -35.00000000000000711, -25.00000000000000711, -7.500000000000000000 ) ) ;
#5779=CARTESIAN_POINT ( 'NONE',  ( -35.00000000000000000, 25.00000000000000000, -7.500000000000000000 ) ) ;
#5781=DIRECTION ( 'NONE',  ( -1.776356839400250465E-15, 0.000000000000000000, 1.000000000000000000 ) ) ;
#5783=CYLINDRICAL_SURFACE ( 'NONE', #5039, 2.500000000000002220 ) ;
#5794=VERTEX_POINT ( 'NONE', #764 ) ;
#5810=CIRCLE ( 'NONE', #10926, 20.00000000000000000 ) ;
#5811=ORIENTED_EDGE ( 'NONE', *, *, #13141, .F. ) ;
#5830=ORIENTED_EDGE ( 'NONE', *, *, #10628, .T. ) ;
#5831=CARTESIAN_POINT ( 'NONE',  ( 35.00000000000000000, 4.286263797015736496E-15, 7.500000000000000000 ) ) ;
#5847=EDGE_CURVE ( 'NONE', #3488, #8713, #12618, .T. ) ;
#5872=LINE ( 'NONE', #10145, #2938 ) ;
#5881=ORIENTED_EDGE ( 'NONE', *, *, #4625, .F. ) ;
#5885=CARTESIAN_POINT ( 'NONE',  ( -35.00000000000000000, -20.00000000000000000, 7.500000000000000000 ) ) ;
#5895=CIRCLE ( 'NONE', #13746, 66.25000000000044054 ) ;
#5909=DIRECTION ( 'NONE',  ( -1.601283208593975514E-16, 1.000000000000000000, 0.000000000000000000 ) ) ;
#5912=CARTESIAN_POINT ( 'NONE',  ( 0.000000000000000000, -20.00000000000000000, 0.000000000000000000 ) ) ;
#5923=FACE_OUTER_BOUND ( 'NONE', #11346, .T. ) ;
#5936=DIRECTION ( 'NONE',  ( 0.000000000000000000, 1.000000000000000000, 0.000000000000000000 ) ) ;
#5939=CIRCLE ( 'NONE', #4127, 15.00000000000000000 ) ;
#5941=VERTEX_POINT ( 'NONE', #8658 ) ;
#5943=EDGE_CURVE ( 'NONE', #13056, #12718, #1862, .T. ) ;
#5952=DIRECTION ( 'NONE',  ( -0.000000000000000000, -0.000000000000000000, 1.000000000000000000 ) ) ;
#5955=DIRECTION ( 'NONE',  ( 1.000000000000000000, 0.000000000000000000, 0.000000000000000000 ) ) ;
#5965=ORIENTED_EDGE ( 'NONE', *, *, #3281, .T. ) ;
#5966=DIRECTION ( 'NONE',  ( 0.000000000000000000, 1.000000000000000000, 0.000000000000000000 ) ) ;
#5969=CARTESIAN_POINT ( 'NONE',  ( 19.84413750617685324, 26.75684992538831963, -2.573597559463546069 ) ) ;
#5975=ORIENTED_EDGE ( 'NONE', *, *, #3614, .T. ) ;
#5981=CARTESIAN_POINT ( 'NONE',  ( -24.37649275748776390, -100.0000000000000000, 7.500000000000000000 ) ) ;
#5982=ORIENTED_EDGE ( 'NONE', *, *, #10986, .F. ) ;
#5991=VERTEX_POINT ( 'NONE', #11815 ) ;
#5997=CARTESIAN_POINT ( 'NONE',  ( -19.18070798040252356, 20.00000000000000000, -4.000000000000000000 ) ) ;
#6000=ORIENTED_EDGE ( 'NONE', *, *, #3097, .F. ) ;
#6010=ORIENTED_EDGE ( 'NONE', *, *, #4983, .F. ) ;
#6018=CIRCLE ( 'NONE', #8470, 22.00000000000000355 ) ;
#6032=ADVANCED_FACE ( 'NONE', ( #11751 ), #10891, .F. ) ;
#6033=CARTESIAN_POINT ( 'NONE',  ( 0.000000000000000000, 0.000000000000000000, 0.000000000000000000 ) ) ;
#6034=CARTESIAN_POINT ( 'NONE',  ( -35.00000000000000000, -35.00000000000000000, 4.000000000000000000 ) ) ;
#6035=CARTESIAN_POINT ( 'NONE',  ( 28.15981099771517648, -27.70535714287384721, 7.500000000000000000 ) ) ;
#6044=DIRECTION ( 'NONE',  ( -1.224646799147353207E-16, 1.000000000000000000, -0.000000000000000000 ) ) ;
#6051=DIRECTION ( 'NONE',  ( -0.000000000000000000, -0.000000000000000000, -1.000000000000000000 ) ) ;
#6053=DIRECTION ( 'NONE',  ( 0.000000000000000000, 0.000000000000000000, 1.000000000000000000 ) ) ;
#6056=VERTEX_POINT ( 'NONE', #9719 ) ;
#6058=CIRCLE ( 'NONE', #7605, 2.500000000000002220 ) ;
#6063=DIRECTION ( 'NONE',  ( 0.000000000000000000, 1.000000000000000000, 0.000000000000000000 ) ) ;
#6072=CARTESIAN_POINT ( 'NONE',  ( -35.00000000000000000, -4.286263797015736496E-15, -4.000000000000000000 ) ) ;
#6074=VECTOR ( 'NONE', #11838, 1000.000000000000000 ) ;
#6080=ORIENTED_EDGE ( 'NONE', *, *, #3373, .F. ) ;
#6095=ORIENTED_EDGE ( 'NONE', *, *, #9620, .F. ) ;
#6099=VERTEX_POINT ( 'NONE', #2493 ) ;
#6102=CARTESIAN_POINT ( 'NONE',  ( -24.37649275748776390, -100.0000000000000000, 7.500000000000000000 ) ) ;
#6128=ORIENTED_EDGE ( 'NONE', *, *, #8733, .F. ) ;
#6130=VERTEX_POINT ( 'NONE', #5536 ) ;
#6156=CYLINDRICAL_SURFACE ( 'NONE', #7476, 22.00000000000000000 ) ;
#6157=CARTESIAN_POINT ( 'NONE',  ( 14.41066181492265130, -21.94006687227777519, 6.364279405527199174 ) ) ;
#6161=DIRECTION ( 'NONE',  ( 0.000000000000000000, -1.000000000000000000, 0.000000000000000000 ) ) ;
#6169=DIRECTION ( 'NONE',  ( -1.000000000000000000, 0.000000000000000000, 0.000000000000000000 ) ) ;
#6172=DIRECTION ( 'NONE',  ( 0.000000000000000000, 0.000000000000000000, 1.000000000000000000 ) ) ;
#6174=DIRECTION ( 'NONE',  ( 0.000000000000000000, -1.000000000000000000, 0.000000000000000000 ) ) ;
#6181=VECTOR ( 'NONE', #8026, 1000.000000000000000 ) ;
#6183=AXIS2_PLACEMENT_3D ( 'NONE', #13306, #3658, #10122 ) ;
#6184=VERTEX_POINT ( 'NONE', #8696 ) ;
#6186=EDGE_LOOP ( 'NONE', ( #10280, #685, #11788, #9803 ) ) ;
#6198=DIRECTION ( 'NONE',  ( -1.000000000000000000, 0.000000000000000000, 0.000000000000000000 ) ) ;
#6213=CARTESIAN_POINT ( 'NONE',  ( 25.00000000000002132, -99.74063674767212717, -4.228074540580630369 ) ) ;
#6214=DIRECTION ( 'NONE',  ( 1.000000000000000000, 0.000000000000000000, 0.000000000000000000 ) ) ;
#6221=ORIENTED_EDGE ( 'NONE', *, *, #7380, .F. ) ;
#6222=ORIENTED_EDGE ( 'NONE', *, *, #8733, .T. ) ;
#6223=PLANE ( 'NONE',  #11746 ) ;
#6240=CIRCLE ( 'NONE', #8909, 2.500000000000002220 ) ;
#6253=LINE ( 'NONE', #4924, #12914 ) ;
#6256=CIRCLE ( 'NONE', #8958, 2.500000000000002220 ) ;
#6267=ADVANCED_FACE ( 'NONE', ( #6594 ), #9824, .T. ) ;
#6277=AXIS2_PLACEMENT_3D ( 'NONE', #3352, #2167, #10654 ) ;
#6279=AXIS2_PLACEMENT_3D ( 'NONE', #12945, #4651, #3308 ) ;
#6283=ORIENTED_EDGE ( 'NONE', *, *, #7820, .T. ) ;
#6286=CARTESIAN_POINT ( 'NONE',  ( -35.00000000000000000, -35.00000000000000000, 7.500000000000000000 ) ) ;
#6300=ORIENTED_EDGE ( 'NONE', *, *, #13630, .T. ) ;
#6308=AXIS2_PLACEMENT_3D ( 'NONE', #97, #8634, #5539 ) ;
#6311=FACE_OUTER_BOUND ( 'NONE', #2015, .T. ) ;
#6312=VERTEX_POINT ( 'NONE', #524 ) ;
#6327=DIRECTION ( 'NONE',  ( -0.000000000000000000, -0.000000000000000000, -1.000000000000000000 ) ) ;
#6328=B_SPLINE_CURVE_WITH_KNOTS ( 'NONE', 3,
 ( #10488, #6157, #5161, #4104, #7395, #5026, #9308, #2006, #11477, #8250, #12543, #12612, #6350, #13756, #2989, #10619 ),
 .UNSPECIFIED., .F., .F.,
 ( 4, 2, 2, 2, 2, 2, 2, 4 ),
 ( 0.000000000000000000, 0.003943481679486459703, 0.005915222519229688253, 0.007886963358972917670, 0.009858704198716145353, 0.01183044503845937477, 0.01380218587820260592, 0.01577392671794583534 ),
 .UNSPECIFIED. ) ;
#6340=EDGE_CURVE ( 'NONE', #12494, #11430, #8145, .T. ) ;
#6350=CARTESIAN_POINT ( 'NONE',  ( 14.85082311557358103, -22.21562007816738316, -5.135570635274604001 ) ) ;
#6353=DIRECTION ( 'NONE',  ( -1.000000000000000000, -2.081668171172168119E-15, 0.000000000000000000 ) ) ;
#6366=DIRECTION ( 'NONE',  ( 0.000000000000000000, 0.000000000000000000, -1.000000000000000000 ) ) ;
#6368=AXIS2_PLACEMENT_3D ( 'NONE', #10683, #4038, #13885 ) ;
#6376=DIRECTION ( 'NONE',  ( -0.000000000000000000, 1.000000000000000000, -0.000000000000000000 ) ) ;
#6379=ORIENTED_EDGE ( 'NONE', *, *, #5228, .F. ) ;
#6381=AXIS2_PLACEMENT_3D ( 'NONE', #3815, #11185, #1775 ) ;
#6391=EDGE_LOOP ( 'NONE', ( #8, #11969 ) ) ;
#6392=COLOUR_RGB ( '', 0.09019608, 0.27058824, 0.51372549) ;
#6394=B_SPLINE_CURVE_WITH_KNOTS ( 'NONE', 3,
 ( #4870, #9148, #8563, #6399 ),
 .UNSPECIFIED., .F., .F.,
 ( 4, 4 ),
 ( 0.03713967652845541478, 0.04074225392669963280 ),
 .UNSPECIFIED. ) ;
#6395=AXIS2_PLACEMENT_3D ( 'NONE', #11847, #8554, #2171 ) ;
#6399=CARTESIAN_POINT ( 'NONE',  ( 24.37649275748779232, -100.0000000000000000, -7.500000000000000000 ) ) ;
#6407=CARTESIAN_POINT ( 'NONE',  ( 25.00000000000001776, -99.86284836912254548, -4.640101051368624496 ) ) ;
#6411=DIRECTION ( 'NONE',  ( -0.000000000000000000, -0.000000000000000000, -1.000000000000000000 ) ) ;
#6413=EDGE_LOOP ( 'NONE', ( #4408, #11902, #13797 ) ) ;
#6423=DIRECTION ( 'NONE',  ( -1.000000000000000000, -1.734723475976805517E-15, 0.000000000000000000 ) ) ;
#6430=EDGE_CURVE ( 'NONE', #4098, #7192, #3893, .T. ) ;
#6448=CARTESIAN_POINT ( 'NONE',  ( 27.38873514654796537, -24.33759740261776017, -4.000000000000000000 ) ) ;
#6452=DIRECTION ( 'NONE',  ( 1.000000000000000000, 2.668805347656626185E-16, -0.000000000000000000 ) ) ;
#6456=ORIENTED_EDGE ( 'NONE', *, *, #4838, .T. ) ;
#6457=VERTEX_POINT ( 'NONE', #10516 ) ;
#6472=AXIS2_PLACEMENT_3D ( 'NONE', #129, #4380, #60 ) ;
#6478=CARTESIAN_POINT ( 'NONE',  ( -35.00000000000000000, 25.00000000000000000, 7.500000000000000000 ) ) ;
#6481=CARTESIAN_POINT ( 'NONE',  ( -35.00000000000000000, -4.286263797015736496E-15, 4.000000000000000000 ) ) ;
#6520=DIRECTION ( 'NONE',  ( 1.000000000000000000, 0.000000000000000000, 0.000000000000000000 ) ) ;
#6526=PLANE ( 'NONE',  #812 ) ;
#6532=EDGE_CURVE ( 'NONE', #5991, #8546, #5040, .T. ) ;
#6537=CARTESIAN_POINT ( 'NONE',  ( -23.64268088454699779, -97.00000000000000000, 0.000000000000000000 ) ) ;
#6546=CARTESIAN_POINT ( 'NONE',  ( 1.387778780781445676E-14, -100.0000000000000000, 0.000000000000000000 ) ) ;
#6566=ORIENTED_EDGE ( 'NONE', *, *, #12510, .T. ) ;
#6567=DIRECTION ( 'NONE',  ( -1.000000000000000000, 0.000000000000000000, 0.000000000000000000 ) ) ;
#6582=DIRECTION ( 'NONE',  ( -2.668805347656626185E-16, 1.000000000000000000, 0.000000000000000000 ) ) ;
#6588=VERTEX_POINT ( 'NONE', #1882 ) ;
#6594=FACE_OUTER_BOUND ( 'NONE', #733, .T. ) ;
#6595=( NAMED_UNIT ( * ) SI_UNIT ( $, .STERADIAN. ) SOLID_ANGLE_UNIT ( ) );
#6604=DIRECTION ( 'NONE',  ( -0.000000000000000000, -0.000000000000000000, -1.000000000000000000 ) ) ;
#6607=DIRECTION ( 'NONE',  ( -0.000000000000000000, -0.000000000000000000, -1.000000000000000000 ) ) ;
#6615=CYLINDRICAL_SURFACE ( 'NONE', #3828, 14.99999999999999645 ) ;
#6617=CARTESIAN_POINT ( 'NONE',  ( 35.00000000000001421, -34.99999999999999289, 7.500000000000000000 ) ) ;
#6618=ORIENTED_EDGE ( 'NONE', *, *, #8007, .T. ) ;
#6621=EDGE_CURVE ( 'NONE', #6312, #10695, #5939, .T. ) ;
#6652=CARTESIAN_POINT ( 'NONE',  ( 15.18222645069203125, 20.00000000000000355, 4.000000000000000000 ) ) ;
#6659=EDGE_CURVE ( 'NONE', #6312, #10078, #8013, .T. ) ;
#6662=VERTEX_POINT ( 'NONE', #6102 ) ;
#6666=CARTESIAN_POINT ( 'NONE',  ( -32.50000000000000000, -3.980102097228898626E-15, -7.500000000000000000 ) ) ;
#6670=CIRCLE ( 'NONE', #2880, 10.00000000000000178 ) ;
#6675=DIRECTION ( 'NONE',  ( 0.000000000000000000, 1.000000000000000000, -0.000000000000000000 ) ) ;
#6682=VERTEX_POINT ( 'NONE', #10501 ) ;
#6685=EDGE_CURVE ( 'NONE', #6758, #5520, #2085, .T. ) ;
#6696=VERTEX_POINT ( 'NONE', #903 ) ;
#6699=DIRECTION ( 'NONE',  ( 0.000000000000000000, 1.000000000000000000, 0.000000000000000000 ) ) ;
#6701=EDGE_CURVE ( 'NONE', #9123, #3490, #4181, .T. ) ;
#6703=EDGE_CURVE ( 'NONE', #7522, #3490, #13803, .T. ) ;
#6710=CIRCLE ( 'NONE', #9417, 10.00000000000000178 ) ;
#6711=CARTESIAN_POINT ( 'NONE',  ( 24.37649275748779232, -100.0000000000000000, 7.500000000000000000 ) ) ;
#6712=VECTOR ( 'NONE', #3309, 1000.000000000000000 ) ;
#6720=AXIS2_PLACEMENT_3D ( 'NONE', #12405, #12472, #2855 ) ;
#6721=CIRCLE ( 'NONE', #5592, 10.00000000000000178 ) ;
#6722=VERTEX_POINT ( 'NONE', #3004 ) ;
#6724=CARTESIAN_POINT ( 'NONE',  ( 19.02348910326480436, 26.95332645987221909, -6.306009631028899776 ) ) ;
#6729=ORIENTED_EDGE ( 'NONE', *, *, #7040, .T. ) ;
#6731=AXIS2_PLACEMENT_3D ( 'NONE', #3398, #1300, #8960 ) ;
#6733=VERTEX_POINT ( 'NONE', #3202 ) ;
#6735=DIRECTION ( 'NONE',  ( 1.000000000000000000, 1.224646799147353207E-16, 0.000000000000000000 ) ) ;
#6740=AXIS2_PLACEMENT_3D ( 'NONE', #7843, #3632, #13206 ) ;
#6741=DIRECTION ( 'NONE',  ( -0.000000000000000000, -0.000000000000000000, -1.000000000000000000 ) ) ;
#6746=FACE_OUTER_BOUND ( 'NONE', #3777, .T. ) ;
#6749=DIRECTION ( 'NONE',  ( 0.000000000000000000, 0.000000000000000000, 1.000000000000000000 ) ) ;
#6757=ORIENTED_EDGE ( 'NONE', *, *, #12611, .F. ) ;
#6758=VERTEX_POINT ( 'NONE', #13771 ) ;
#6765=EDGE_CURVE ( 'NONE', #9535, #10692, #65, .T. ) ;
#6783=CARTESIAN_POINT ( 'NONE',  ( 25.00000000000000711, -34.99999999999999289, 7.500000000000000000 ) ) ;
#6785=DIRECTION ( 'NONE',  ( -0.000000000000000000, -0.000000000000000000, -1.000000000000000000 ) ) ;
#6789=EDGE_CURVE ( 'NONE', #2423, #5794, #8600, .T. ) ;
#6790=AXIS2_PLACEMENT_3D ( 'NONE', #6537, #231, #13077 ) ;
#6791=DIRECTION ( 'NONE',  ( 0.000000000000000000, -0.000000000000000000, -1.000000000000000000 ) ) ;
#6797=CARTESIAN_POINT ( 'NONE',  ( -31.93204061526060045, -3.910547132972217398E-15, 0.000000000000000000 ) ) ;
#6800=LINE ( 'NONE', #510, #8068 ) ;
#6811=CARTESIAN_POINT ( 'NONE',  ( -60.00000000000001421, 20.00000000000000000, -4.000000000000000000 ) ) ;
#6812=( LENGTH_UNIT ( ) NAMED_UNIT ( * ) SI_UNIT ( .MILLI., .METRE. ) );
#6822=EDGE_LOOP ( 'NONE', ( #13359, #9339, #12253, #13530, #1092, #5418 ) ) ;
#6825=CARTESIAN_POINT ( 'NONE',  ( -32.50000000000000000, -3.980102097228898626E-15, 7.500000000000000000 ) ) ;
#6827=ORIENTED_EDGE ( 'NONE', *, *, #11484, .T. ) ;
#6829=DIRECTION ( 'NONE',  ( -0.000000000000000000, 0.000000000000000000, -1.000000000000000000 ) ) ;
#6830=CARTESIAN_POINT ( 'NONE',  ( -18.54049621773915746, -20.00000000000000000, -7.500000000000000000 ) ) ;
#6831=CARTESIAN_POINT ( 'NONE',  ( 19.18070798040252356, 20.00000000000000000, -4.000000000000000000 ) ) ;
#6833=AXIS2_PLACEMENT_3D ( 'NONE', #7577, #8631, #4414 ) ;
#6836=ORIENTED_EDGE ( 'NONE', *, *, #12173, .T. ) ;
#6840=DIRECTION ( 'NONE',  ( 0.000000000000000000, -0.000000000000000000, 1.000000000000000000 ) ) ;
#6850=CIRCLE ( 'NONE', #598, 10.00000000000000178 ) ;
#6858=CARTESIAN_POINT ( 'NONE',  ( 25.00000000000001776, -100.0000000000000000, -7.500000000000000000 ) ) ;
#6875=CARTESIAN_POINT ( 'NONE',  ( -35.00000000000000000, -4.286263797015736496E-15, 7.500000000000000000 ) ) ;
#6879=ORIENTED_EDGE ( 'NONE', *, *, #4359, .F. ) ;
#6887=PLANE ( 'NONE',  #5336 ) ;
#6889=CARTESIAN_POINT ( 'NONE',  ( 15.68886946032145957, -16.65327071804363612, 0.6902218057983463551 ) ) ;
#6891=LINE ( 'NONE', #6825, #8099 ) ;
#6897=ORIENTED_EDGE ( 'NONE', *, *, #5734, .T. ) ;
#6909=CARTESIAN_POINT ( 'NONE',  ( -24.99999999999998934, -100.0000000000000000, 7.500000000000000000 ) ) ;
#6914=DIRECTION ( 'NONE',  ( 0.000000000000000000, 1.000000000000000000, 0.000000000000000000 ) ) ;
#6920=EDGE_CURVE ( 'NONE', #10078, #618, #5435, .T. ) ;
#6931=DIRECTION ( 'NONE',  ( 0.000000000000000000, 1.000000000000000000, 0.000000000000000000 ) ) ;
#6940=ORIENTED_EDGE ( 'NONE', *, *, #12701, .T. ) ;
#6943=ORIENTED_EDGE ( 'NONE', *, *, #573, .F. ) ;
#6949=DIRECTION ( 'NONE',  ( -0.000000000000000000, -0.000000000000000000, -1.000000000000000000 ) ) ;
#6951=FACE_OUTER_BOUND ( 'NONE', #47, .T. ) ;
#6958=CARTESIAN_POINT ( 'NONE',  ( -28.15981099771517648, -27.70535714287384366, -4.000000000000000000 ) ) ;
#6971=DIRECTION ( 'NONE',  ( -1.000000000000000000, 0.000000000000000000, 0.000000000000000000 ) ) ;
#6972=CIRCLE ( 'NONE', #12357, 66.25000000000044054 ) ;
#6976=ORIENTED_EDGE ( 'NONE', *, *, #9107, .T. ) ;
#6995=CYLINDRICAL_SURFACE ( 'NONE', #1002, 25.50000000002550138 ) ;
#7007=CARTESIAN_POINT ( 'NONE',  ( 37.50000000000000711, 4.592425496802575156E-15, -7.500000000000000000 ) ) ;
#7017=DIRECTION ( 'NONE',  ( 1.000000000000000000, 0.000000000000000000, 0.000000000000000000 ) ) ;
#7029=ORIENTED_EDGE ( 'NONE', *, *, #12196, .T. ) ;
#7033=AXIS2_PLACEMENT_3D ( 'NONE', #9059, #521, #7017 ) ;
#7035=CARTESIAN_POINT ( 'NONE',  ( -35.00000000000000000, -35.00000000000000000, 7.500000000000000000 ) ) ;
#7036=DIRECTION ( 'NONE',  ( -0.000000000000000000, -0.000000000000000000, -1.000000000000000000 ) ) ;
#7038=LINE ( 'NONE', #6830, #8856 ) ;
#7040=EDGE_CURVE ( 'NONE', #10943, #1175, #12823, .T. ) ;
#7055=VERTEX_POINT ( 'NONE', #2275 ) ;
#7064=CARTESIAN_POINT ( 'NONE',  ( -37.50000000000000711, -4.286263797015736496E-15, -4.000000000000000000 ) ) ;
#7065=VECTOR ( 'NONE', #3040, 1000.000000000000000 ) ;
#7073=DIRECTION ( 'NONE',  ( 1.000000000000000000, 0.000000000000000000, 0.000000000000000000 ) ) ;
#7094=DIRECTION ( 'NONE',  ( 0.000000000000000000, 0.000000000000000000, 1.000000000000000000 ) ) ;
#7119=VECTOR ( 'NONE', #1883, 1000.000000000000000 ) ;
#7135=EDGE_CURVE ( 'NONE', #3214, #8349, #1169, .T. ) ;
#7138=EDGE_CURVE ( 'NONE', #470, #1947, #9497, .T. ) ;
#7141=ORIENTED_EDGE ( 'NONE', *, *, #9869, .T. ) ;
#7146=DIRECTION ( 'NONE',  ( -1.000000000000000000, 0.000000000000000000, 0.000000000000000000 ) ) ;
#7154=FACE_OUTER_BOUND ( 'NONE', #1164, .T. ) ;
#7159=CARTESIAN_POINT ( 'NONE',  ( -14.37641089434894326, -21.93614314624077721, 6.343488216808987445 ) ) ;
#7161=AXIS2_PLACEMENT_3D ( 'NONE', #4218, #13673, #2976 ) ;
#7164=CIRCLE ( 'NONE', #1824, 25.00000000000000711 ) ;
#7172=DIRECTION ( 'NONE',  ( -0.000000000000000000, -0.000000000000000000, -1.000000000000000000 ) ) ;
#7181=CARTESIAN_POINT ( 'NONE',  ( -18.99432778721694604, 26.96223687785629508, -6.295342420724992394 ) ) ;
#7187=ORIENTED_EDGE ( 'NONE', *, *, #4727, .T. ) ;
#7189=DIRECTION ( 'NONE',  ( -1.000000000000000000, 0.000000000000000000, 0.000000000000000000 ) ) ;
#7192=VERTEX_POINT ( 'NONE', #10346 ) ;
#7194=CARTESIAN_POINT ( 'NONE',  ( -15.34996685542352424, -16.25414556851945491, -3.363331797608928309 ) ) ;
#7196=EDGE_CURVE ( 'NONE', #12718, #6056, #2915, .T. ) ;
#7201=CARTESIAN_POINT ( 'NONE',  ( 13.79311422413708499, -100.0000000000000000, 7.500000000000000000 ) ) ;
#7208=ADVANCED_FACE ( 'NONE', ( #4944 ), #10063, .F. ) ;
#7213=ADVANCED_FACE ( 'NONE', ( #4874 ), #8035, .F. ) ;
#7217=ORIENTED_EDGE ( 'NONE', *, *, #801, .T. ) ;
#7219=CARTESIAN_POINT ( 'NONE',  ( -35.00000000000000000, -4.286263797015736496E-15, 4.000000000000000000 ) ) ;
#7225=ORIENTED_EDGE ( 'NONE', *, *, #12861, .F. ) ;
#7232=VECTOR ( 'NONE', #8123, 1000.000000000000000 ) ;
#7240=FACE_OUTER_BOUND ( 'NONE', #11558, .T. ) ;
#7244=CARTESIAN_POINT ( 'NONE',  ( 22.00000000000000711, -100.0000000000000000, 2.694222958124176809E-15 ) ) ;
#7248=CARTESIAN_POINT ( 'NONE',  ( 25.00000000000001776, -99.15310334213020838, 3.061571689641656246E-15 ) ) ;
#7250=AXIS2_PLACEMENT_3D ( 'NONE', #7788, #12296, #6749 ) ;
#7252=ORIENTED_EDGE ( 'NONE', *, *, #8750, .F. ) ;
#7255=ORIENTED_EDGE ( 'NONE', *, *, #9852, .T. ) ;
#7261=PLANE ( 'NONE',  #227 ) ;
#7268=CARTESIAN_POINT ( 'NONE',  ( 1.922734475756564121E-15, -100.0000000000000000, -15.70031846811053455 ) ) ;
#7273=ORIENTED_EDGE ( 'NONE', *, *, #4649, .F. ) ;
#7282=ADVANCED_FACE ( 'NONE', ( #613 ), #13541, .F. ) ;
#7285=EDGE_CURVE ( 'NONE', #5648, #9044, #7603, .T. ) ;
#7291=EDGE_LOOP ( 'NONE', ( #1000, #9072, #7451, #11184, #10709, #10787, #9235 ) ) ;
#7292=DIRECTION ( 'NONE',  ( -1.000000000000000000, 0.000000000000000000, 0.000000000000000000 ) ) ;
#7298=FACE_OUTER_BOUND ( 'NONE', #10434, .T. ) ;
#7305=ORIENTED_EDGE ( 'NONE', *, *, #867, .F. ) ;
#7315=VECTOR ( 'NONE', #1381, 1000.000000000000000 ) ;
#7316=CARTESIAN_POINT ( 'NONE',  ( -22.42156014662057473, -97.00000000000000000, 7.500000000000000000 ) ) ;
#7319=ORIENTED_EDGE ( 'NONE', *, *, #10303, .T. ) ;
#7329=CYLINDRICAL_SURFACE ( 'NONE', #13717, 66.25000000000044054 ) ;
#7332=CARTESIAN_POINT ( 'NONE',  ( 22.42156014662059249, -97.00000000000000000, -7.500000000000000000 ) ) ;
#7334=ORIENTED_EDGE ( 'NONE', *, *, #1742, .T. ) ;
#7342=AXIS2_PLACEMENT_3D ( 'NONE', #10992, #7559, #6520 ) ;
#7348=DIRECTION ( 'NONE',  ( 1.000000000000000000, 2.081668171172168119E-15, 0.000000000000000000 ) ) ;
#7357=CARTESIAN_POINT ( 'NONE',  ( -24.99999999999999645, -99.74063674767198506, 4.228074540580154306 ) ) ;
#7358=CARTESIAN_POINT ( 'NONE',  ( 1.187907395172932673E-14, -97.00000000000000000, 0.000000000000000000 ) ) ;
#7372=EDGE_CURVE ( 'NONE', #9123, #13392, #12555, .T. ) ;
#7375=EDGE_CURVE ( 'NONE', #2284, #10314, #10083, .T. ) ;
#7380=EDGE_CURVE ( 'NONE', #4069, #13581, #9561, .T. ) ;
#7388=CIRCLE ( 'NONE', #11873, 2.000000000000001776 ) ;
#7393=DIRECTION ( 'NONE',  ( 0.000000000000000000, 1.000000000000000000, -0.000000000000000000 ) ) ;
#7395=CARTESIAN_POINT ( 'NONE',  ( 15.49340857339600142, -22.63585399314533575, 2.623848604783063365 ) ) ;
#7405=ORIENTED_EDGE ( 'NONE', *, *, #5693, .F. ) ;
#7419=DIRECTION ( 'NONE',  ( -0.000000000000000000, -0.000000000000000000, -1.000000000000000000 ) ) ;
#7428=DIRECTION ( 'NONE',  ( 1.000000000000000000, 0.000000000000000000, 0.000000000000000000 ) ) ;
#7432=DIRECTION ( 'NONE',  ( 0.000000000000000000, 1.000000000000000000, 0.000000000000000000 ) ) ;
#7435=ORIENTED_EDGE ( 'NONE', *, *, #12611, .T. ) ;
#7445=CARTESIAN_POINT ( 'NONE',  ( 0.000000000000000000, 40.00000000000000000, 20.00000000000000000 ) ) ;
#7451=ORIENTED_EDGE ( 'NONE', *, *, #8245, .T. ) ;
#7458=ADVANCED_FACE ( 'NONE', ( #6746 ), #7717, .T. ) ;
#7459=ORIENTED_EDGE ( 'NONE', *, *, #5306, .T. ) ;
#7470=FACE_OUTER_BOUND ( 'NONE', #12508, .T. ) ;
#7472=DIRECTION ( 'NONE',  ( -0.000000000000000000, -0.000000000000000000, -1.000000000000000000 ) ) ;
#7476=AXIS2_PLACEMENT_3D ( 'NONE', #690, #2718, #9376 ) ;
#7478=ORIENTED_EDGE ( 'NONE', *, *, #6703, .T. ) ;
#7482=AXIS2_PLACEMENT_3D ( 'NONE', #4433, #8715, #4373 ) ;
#7487=ORIENTED_EDGE ( 'NONE', *, *, #2929, .T. ) ;
#7494=VERTEX_POINT ( 'NONE', #4417 ) ;
#7506=CARTESIAN_POINT ( 'NONE',  ( -26.79177319725820894, -26.24642857144861807, -4.000000000000000000 ) ) ;
#7512=LINE ( 'NONE', #2182, #13700 ) ;
#7518=DIRECTION ( 'NONE',  ( -0.000000000000000000, -0.000000000000000000, 1.000000000000000000 ) ) ;
#7522=VERTEX_POINT ( 'NONE', #6666 ) ;
#7557=CARTESIAN_POINT ( 'NONE',  ( 30.72062512117249611, 25.13835616439071785, 0.000000000000000000 ) ) ;
#7558=CIRCLE ( 'NONE', #3305, 25.00000000000000355 ) ;
#7559=DIRECTION ( 'NONE',  ( 0.000000000000000000, 0.000000000000000000, 1.000000000000000000 ) ) ;
#7565=LINE ( 'NONE', #3155, #141 ) ;
#7568=ORIENTED_EDGE ( 'NONE', *, *, #3281, .F. ) ;
#7571=CIRCLE ( 'NONE', #13678, 25.00000000000000711 ) ;
#7577=CARTESIAN_POINT ( 'NONE',  ( 1.653273178848927024E-14, -135.0000000000000000, 0.000000000000000000 ) ) ;
#7582=CIRCLE ( 'NONE', #13688, 25.50418395392908977 ) ;
#7586=CARTESIAN_POINT ( 'NONE',  ( -24.99999999999998934, -100.0000000000065938, -5.046127144261280506 ) ) ;
#7589=DIRECTION ( 'NONE',  ( -1.224646799147353207E-16, 1.000000000000000000, 0.000000000000000000 ) ) ;
#7603=CIRCLE ( 'NONE', #466, 2.500000000000002220 ) ;
#7605=AXIS2_PLACEMENT_3D ( 'NONE', #194, #4445, #8727 ) ;
#7609=EDGE_CURVE ( 'NONE', #10258, #6662, #5258, .T. ) ;
#7621=CIRCLE ( 'NONE', #11886, 2.500000000000002220 ) ;
#7623=EDGE_CURVE ( 'NONE', #618, #10695, #2755, .T. ) ;
#7626=EDGE_LOOP ( 'NONE', ( #9584, #12181 ) ) ;
#7627=CARTESIAN_POINT ( 'NONE',  ( 22.00000000000000000, 2.694222958124176809E-15, 2.694222958124176809E-15 ) ) ;
#7628=ORIENTED_EDGE ( 'NONE', *, *, #966, .T. ) ;
#7631=EDGE_CURVE ( 'NONE', #4855, #9446, #9345, .T. ) ;
#7636=DIRECTION ( 'NONE',  ( 0.000000000000000000, 1.000000000000000000, 0.000000000000000000 ) ) ;
#7639=ORIENTED_EDGE ( 'NONE', *, *, #979, .F. ) ;
#7642=ADVANCED_FACE ( 'NONE', ( #7298 ), #9609, .F. ) ;
#7657=ORIENTED_EDGE ( 'NONE', *, *, #7372, .T. ) ;
#7662=CARTESIAN_POINT ( 'NONE',  ( -6.999999999999999112, -20.00000000000000355, 7.500000000000000000 ) ) ;
#7680=VERTEX_POINT ( 'NONE', #6652 ) ;
#7686=LINE ( 'NONE', #10773, #2419 ) ;
#7687=CIRCLE ( 'NONE', #11510, 25.50000000002550138 ) ;
#7688=EDGE_LOOP ( 'NONE', ( #3997, #9985, #4627, #11062 ) ) ;
#7690=VERTEX_POINT ( 'NONE', #3218 ) ;
#7700=ADVANCED_FACE ( 'NONE', ( #1318, #9887 ), #11980, .T. ) ;
#7706=EDGE_CURVE ( 'NONE', #7751, #6696, #9424, .T. ) ;
#7709=CYLINDRICAL_SURFACE ( 'NONE', #4446, 2.000000000000001776 ) ;
#7717=CYLINDRICAL_SURFACE ( 'NONE', #1121, 25.00000000000000355 ) ;
#7719=CARTESIAN_POINT ( 'NONE',  ( -21.99999999999999289, -97.00000000000000000, 7.500000000000000000 ) ) ;
#7722=EDGE_LOOP ( 'NONE', ( #4062, #13596, #9405, #13337 ) ) ;
#7727=CARTESIAN_POINT ( 'NONE',  ( -24.99999999999998579, -99.51472204732199600, -3.411167378945827000 ) ) ;
#7730=EDGE_LOOP ( 'NONE', ( #13457, #3095, #10484 ) ) ;
#7734=CARTESIAN_POINT ( 'NONE',  ( -24.37649275748776390, -100.0000000000000000, -7.500000000000000000 ) ) ;
#7746=CARTESIAN_POINT ( 'NONE',  ( 37.50000000000000711, 4.592425496802575156E-15, -4.000000000000000000 ) ) ;
#7747=AXIS2_PLACEMENT_3D ( 'NONE', #12097, #1506, #10064 ) ;
#7748=ORIENTED_EDGE ( 'NONE', *, *, #6532, .T. ) ;
#7751=VERTEX_POINT ( 'NONE', #7007 ) ;
#7754=FACE_OUTER_BOUND ( 'NONE', #7759, .T. ) ;
#7758=EDGE_CURVE ( 'NONE', #5016, #13646, #3916, .T. ) ;
#7759=EDGE_LOOP ( 'NONE', ( #253, #9146, #3280, #1004 ) ) ;
#7763=CARTESIAN_POINT ( 'NONE',  ( 22.00000000000001066, -97.00000000000000000, 0.000000000000000000 ) ) ;
#7766=FACE_OUTER_BOUND ( 'NONE', #3401, .T. ) ;
#7769=LINE ( 'NONE', #9892, #13140 ) ;
#7771=ORIENTED_EDGE ( 'NONE', *, *, #5225, .T. ) ;
#7775=EDGE_CURVE ( 'NONE', #4007, #13581, #4246, .T. ) ;
#7786=DIRECTION ( 'NONE',  ( 0.000000000000000000, 1.000000000000000000, 0.000000000000000000 ) ) ;
#7788=CARTESIAN_POINT ( 'NONE',  ( 0.000000000000000000, -20.00000000000000000, 0.000000000000000000 ) ) ;
#7796=EDGE_CURVE ( 'NONE', #3488, #8612, #6800, .T. ) ;
#7797=PLANE ( 'NONE',  #12337 ) ;
#7804=CARTESIAN_POINT ( 'NONE',  ( -37.50000000000000711, -4.286263797015736496E-15, -7.500000000000000000 ) ) ;
#7807=EDGE_CURVE ( 'NONE', #3663, #3080, #9855, .T. ) ;
#7811=CARTESIAN_POINT ( 'NONE',  ( -20.00023673640403743, 26.72039747452867076, -1.279702169315401150 ) ) ;
#7820=EDGE_CURVE ( 'NONE', #13581, #4007, #3811, .T. ) ;
#7825=EDGE_CURVE ( 'NONE', #12409, #9553, #11221, .T. ) ;
#7828=LINE ( 'NONE', #6783, #1721 ) ;
#7830=DIRECTION ( 'NONE',  ( 0.000000000000000000, 0.000000000000000000, 1.000000000000000000 ) ) ;
#7832=UNCERTAINTY_MEASURE_WITH_UNIT (LENGTH_MEASURE( 1.000000000000000082E-05 ), #6812, 'distance_accuracy_value', 'NONE');
#7843=CARTESIAN_POINT ( 'NONE',  ( -60.00000000000001421, 20.00000000000000000, 4.000000000000000000 ) ) ;
#7845=CARTESIAN_POINT ( 'NONE',  ( 0.000000000000000000, 40.00000000000000000, 0.000000000000000000 ) ) ;
#7852=AXIS2_PLACEMENT_3D ( 'NONE', #8900, #3779, #12203 ) ;
#7854=ORIENTED_EDGE ( 'NONE', *, *, #7040, .F. ) ;
#7860=( LENGTH_UNIT ( ) NAMED_UNIT ( * ) SI_UNIT ( .MILLI., .METRE. ) );
#7863=CARTESIAN_POINT ( 'NONE',  ( -28.15981099771517648, -27.70535714287384366, 7.500000000000000000 ) ) ;
#7880=LINE ( 'NONE', #1773, #6181 ) ;
#7881=CARTESIAN_POINT ( 'NONE',  ( 7.000000000000007994, -35.00000000000000000, 7.500000000000000000 ) ) ;
#7894=EDGE_CURVE ( 'NONE', #7680, #2431, #11494, .T. ) ;
#7900=EDGE_CURVE ( 'NONE', #5991, #5794, #8972, .T. ) ;
#7902=ORIENTED_EDGE ( 'NONE', *, *, #12884, .T. ) ;
#7903=DIRECTION ( 'NONE',  ( 1.000000000000000000, 0.000000000000000000, 0.000000000000000000 ) ) ;
#7913=ORIENTED_EDGE ( 'NONE', *, *, #1639, .F. ) ;
#7922=DIRECTION ( 'NONE',  ( -0.000000000000000000, -0.000000000000000000, -1.000000000000000000 ) ) ;
#7924=AXIS2_PLACEMENT_3D ( 'NONE', #2324, #6607, #1276 ) ;
#7926=CARTESIAN_POINT ( 'NONE',  ( 35.00000000000001421, -135.0000000000000000, 4.286263797015737285E-15 ) ) ;
#7930=B_SPLINE_CURVE_WITH_KNOTS ( 'NONE', 3,
 ( #8710, #3515, #7727, #11024, #5629, #2268, #1285, #12947 ),
 .UNSPECIFIED., .F., .F.,
 ( 4, 2, 2, 4 ),
 ( 0.02189346042269429971, 0.02442701477284284911, 0.02569379194791712034, 0.02696056912299139158 ),
 .UNSPECIFIED. ) ;
#7937=ORIENTED_EDGE ( 'NONE', *, *, #7894, .T. ) ;
#7944=CARTESIAN_POINT ( 'NONE',  ( 15.34996685542352424, -16.25414556851945491, 3.363331797608928309 ) ) ;
#7954=EDGE_LOOP ( 'NONE', ( #9221, #7771, #10633, #5383 ) ) ;
#7976=DIRECTION ( 'NONE',  ( -1.000000000000000000, 0.000000000000000000, 0.000000000000000000 ) ) ;
#7980=VECTOR ( 'NONE', #5360, 1000.000000000000000 ) ;
#7989=VERTEX_POINT ( 'NONE', #3527 ) ;
#7998=CARTESIAN_POINT ( 'NONE',  ( 0.000000000000000000, 40.00000000000000000, 0.000000000000000000 ) ) ;
#8007=EDGE_CURVE ( 'NONE', #2559, #5941, #5391, .T. ) ;
#8013=LINE ( 'NONE', #2680, #4818 ) ;
#8019=CARTESIAN_POINT ( 'NONE',  ( 15.18222645069203303, -16.04698886238941924, -4.000000000000000000 ) ) ;
#8026=DIRECTION ( 'NONE',  ( 1.000000000000000000, 1.224646799147353207E-16, 0.000000000000000000 ) ) ;
#8032=DIRECTION ( 'NONE',  ( -1.000000000000000000, 0.000000000000000000, 0.000000000000000000 ) ) ;
#8034=CARTESIAN_POINT ( 'NONE',  ( -34.24999999999972999, -135.0000000000000000, -4.194415287079653581E-15 ) ) ;
#8035=PLANE ( 'NONE',  #9400 ) ;
#8049=CARTESIAN_POINT ( 'NONE',  ( -35.00000000000000000, 25.00000000000000000, 7.500000000000000000 ) ) ;
#8057=ORIENTED_EDGE ( 'NONE', *, *, #4916, .F. ) ;
#8067=EDGE_CURVE ( 'NONE', #12537, #11430, #10974, .T. ) ;
#8068=VECTOR ( 'NONE', #1534, 1000.000000000000000 ) ;
#8078=DIRECTION ( 'NONE',  ( -0.000000000000000000, -0.000000000000000000, -1.000000000000000000 ) ) ;
#8091=ORIENTED_EDGE ( 'NONE', *, *, #8570, .F. ) ;
#8093=DIRECTION ( 'NONE',  ( -0.000000000000000000, -0.000000000000000000, -1.000000000000000000 ) ) ;
#8094=VERTEX_POINT ( 'NONE', #3679 ) ;
#8096=CARTESIAN_POINT ( 'NONE',  ( -35.00000000000000000, -4.286263797015736496E-15, 4.000000000000000000 ) ) ;
#8098=VECTOR ( 'NONE', #11148, 1000.000000000000000 ) ;
#8099=VECTOR ( 'NONE', #8093, 1000.000000000000000 ) ;
#8107=CARTESIAN_POINT ( 'NONE',  ( 28.79177319725820183, -26.24642857144861807, -4.000000000000000000 ) ) ;
#8123=DIRECTION ( 'NONE',  ( -0.000000000000000000, -0.000000000000000000, -1.000000000000000000 ) ) ;
#8133=DIRECTION ( 'NONE',  ( -0.000000000000000000, -0.000000000000000000, -1.000000000000000000 ) ) ;
#8145=LINE ( 'NONE', #6811, #10803 ) ;
#8149=DIRECTION ( 'NONE',  ( -1.000000000000000000, -1.224646799147353207E-16, 0.000000000000000000 ) ) ;
#8151=FACE_OUTER_BOUND ( 'NONE', #4115, .T. ) ;
#8153=EDGE_CURVE ( 'NONE', #12537, #5686, #5872, .T. ) ;
#8159=DIRECTION ( 'NONE',  ( 1.000000000000000000, 0.000000000000000000, 0.000000000000000000 ) ) ;
#8172=DIRECTION ( 'NONE',  ( 0.000000000000000000, 0.000000000000000000, 1.000000000000000000 ) ) ;
#8190=EDGE_CURVE ( 'NONE', #9553, #12643, #5171, .T. ) ;
#8193=AXIS2_PLACEMENT_3D ( 'NONE', #1409, #10931, #382 ) ;
#8195=ORIENTED_EDGE ( 'NONE', *, *, #4210, .T. ) ;
#8197=DIRECTION ( 'NONE',  ( 5.337610695313252124E-17, -1.000000000000000000, 0.000000000000000000 ) ) ;
#8198=CIRCLE ( 'NONE', #2362, 1.999999999999998224 ) ;
#8208=ORIENTED_EDGE ( 'NONE', *, *, #9849, .T. ) ;
#8213=EDGE_LOOP ( 'NONE', ( #6827, #91 ) ) ;
#8215=CARTESIAN_POINT ( 'NONE',  ( -31.93204061526058624, -132.0000000000000000, 0.000000000000000000 ) ) ;
#8217=FACE_BOUND ( 'NONE', #9335, .T. ) ;
#8221=AXIS2_PLACEMENT_3D ( 'NONE', #4742, #9020, #4813 ) ;
#8229=VERTEX_POINT ( 'NONE', #7316 ) ;
#8239=ORIENTED_EDGE ( 'NONE', *, *, #452, .T. ) ;
#8245=EDGE_CURVE ( 'NONE', #2481, #12788, #1551, .T. ) ;
#8250=CARTESIAN_POINT ( 'NONE',  ( 15.49491024508755999, -22.63688244086936763, -2.616826951557488457 ) ) ;
#8261=CARTESIAN_POINT ( 'NONE',  ( -21.99999999999999289, -100.0000000000000000, 7.500000000000000000 ) ) ;
#8262=ADVANCED_FACE ( 'NONE', ( #9432 ), #9564, .T. ) ;
#8263=ORIENTED_EDGE ( 'NONE', *, *, #4727, .F. ) ;
#8272=DIRECTION ( 'NONE',  ( 0.000000000000000000, 0.000000000000000000, 1.000000000000000000 ) ) ;
#8273=VERTEX_POINT ( 'NONE', #10674 ) ;
#8275=ORIENTED_EDGE ( 'NONE', *, *, #4210, .F. ) ;
#8279=AXIS2_PLACEMENT_3D ( 'NONE', #7035, #6829, #11314 ) ;
#8285=DIRECTION ( 'NONE',  ( 1.000000000000000000, 0.000000000000000000, 0.000000000000000000 ) ) ;
#8286=DIRECTION ( 'NONE',  ( -0.000000000000000000, 1.000000000000000000, -0.000000000000000000 ) ) ;
#8297=CARTESIAN_POINT ( 'NONE',  ( -24.37649275748776390, -100.0000000000000000, -7.500000000000000000 ) ) ;
#8321=DIRECTION ( 'NONE',  ( 0.000000000000000000, 0.000000000000000000, 1.000000000000000000 ) ) ;
#8343=EDGE_CURVE ( 'NONE', #10920, #4208, #4499, .T. ) ;
#8347=ORIENTED_EDGE ( 'NONE', *, *, #10772, .T. ) ;
#8349=VERTEX_POINT ( 'NONE', #8639 ) ;
#8361=VERTEX_POINT ( 'NONE', #240 ) ;
#8377=DIRECTION ( 'NONE',  ( 0.000000000000000000, 0.000000000000000000, 1.000000000000000000 ) ) ;
#8381=CARTESIAN_POINT ( 'NONE',  ( 35.00000000000000000, 4.286263797015736496E-15, 4.000000000000000000 ) ) ;
#8386=CARTESIAN_POINT ( 'NONE',  ( 0.000000000000000000, 40.00000000000000000, 0.000000000000000000 ) ) ;
#8387=CARTESIAN_POINT ( 'NONE',  ( -60.00000000000001421, 20.00000000000000000, -4.000000000000000000 ) ) ;
#8396=ADVANCED_FACE ( 'NONE', ( #1275 ), #174, .F. ) ;
#8399=EDGE_CURVE ( 'NONE', #5520, #9444, #5412, .T. ) ;
#8400=DIRECTION ( 'NONE',  ( -0.000000000000000000, -0.000000000000000000, -1.000000000000000000 ) ) ;
#8410=ADVANCED_FACE ( 'NONE', ( #8777 ), #4420, .T. ) ;
#8416=ORIENTED_EDGE ( 'NONE', *, *, #7138, .T. ) ;
#8417=DIRECTION ( 'NONE',  ( -0.000000000000000000, -0.000000000000000000, -1.000000000000000000 ) ) ;
#8418=EDGE_LOOP ( 'NONE', ( #13681, #1372 ) ) ;
#8423=AXIS2_PLACEMENT_3D ( 'NONE', #11683, #711, #3784 ) ;
#8424=CARTESIAN_POINT ( 'NONE',  ( -13.79311422413708499, -21.62638421600851046, -7.500000000000000000 ) ) ;
#8443=FACE_OUTER_BOUND ( 'NONE', #8987, .T. ) ;
#8444=CARTESIAN_POINT ( 'NONE',  ( -35.00000000000000000, -4.286263797015736496E-15, 7.500000000000000000 ) ) ;
#8457=CARTESIAN_POINT ( 'NONE',  ( 32.50000000000000000, 4.286263797015736496E-15, 7.500000000000000000 ) ) ;
#8460=ORIENTED_EDGE ( 'NONE', *, *, #12173, .F. ) ;
#8468=EDGE_CURVE ( 'NONE', #13392, #9123, #11160, .T. ) ;
#8470=AXIS2_PLACEMENT_3D ( 'NONE', #10023, #2738, #4690 ) ;
#8488=CARTESIAN_POINT ( 'NONE',  ( -35.00000000000000711, -25.00000000000000711, 7.500000000000000000 ) ) ;
#8492=EDGE_LOOP ( 'NONE', ( #6566, #12774, #9156, #4327, #3927, #2242, #11068, #1330 ) ) ;
#8494=EDGE_CURVE ( 'NONE', #8894, #1175, #11388, .T. ) ;
#8503=AXIS2_PLACEMENT_3D ( 'NONE', #10743, #3444, #12009 ) ;
#8518=LINE ( 'NONE', #9643, #5701 ) ;
#8519=CARTESIAN_POINT ( 'NONE',  ( 1.387778780781445676E-14, -100.0000000000000000, 0.000000000000000000 ) ) ;
#8522=DIRECTION ( 'NONE',  ( -0.000000000000000000, -0.000000000000000000, -1.000000000000000000 ) ) ;
#8524=LINE ( 'NONE', #12827, #2146 ) ;
#8544=EDGE_CURVE ( 'NONE', #2431, #9931, #5712, .T. ) ;
#8546=VERTEX_POINT ( 'NONE', #6958 ) ;
#8554=DIRECTION ( 'NONE',  ( -0.000000000000000000, -0.000000000000000000, -1.000000000000000000 ) ) ;
#8563=CARTESIAN_POINT ( 'NONE',  ( 23.75221630157310315, -98.98132178242397572, -7.500000000000000000 ) ) ;
#8570=EDGE_CURVE ( 'NONE', #5648, #1545, #4926, .T. ) ;
#8587=CYLINDRICAL_SURFACE ( 'NONE', #6368, 25.00000000000000711 ) ;
#8594=DIRECTION ( 'NONE',  ( -1.000000000000000000, 0.000000000000000000, 0.000000000000000000 ) ) ;
#8597=CIRCLE ( 'NONE', #7033, 25.50000000002550138 ) ;
#8600=LINE ( 'NONE', #8886, #13575 ) ;
#8604=CARTESIAN_POINT ( 'NONE',  ( -19.84413750617685324, 26.75684992538831253, 2.573597559463546069 ) ) ;
#8605=CARTESIAN_POINT ( 'NONE',  ( 22.42156014662059249, -97.00000000000000000, 7.500000000000000000 ) ) ;
#8611=CIRCLE ( 'NONE', #12668, 25.00000000000000711 ) ;
#8612=VERTEX_POINT ( 'NONE', #9122 ) ;
#8623=STYLED_ITEM ( 'NONE', ( #5473 ), #11412 ) ;
#8631=DIRECTION ( 'NONE',  ( -1.224646799147353207E-16, 1.000000000000000000, -0.000000000000000000 ) ) ;
#8634=DIRECTION ( 'NONE',  ( -0.000000000000000000, -0.000000000000000000, -1.000000000000000000 ) ) ;
#8639=CARTESIAN_POINT ( 'NONE',  ( -13.79311422413708499, -20.00000000000000355, -7.500000000000000000 ) ) ;
#8658=CARTESIAN_POINT ( 'NONE',  ( -18.54049621773915746, 27.07720798311999388, -7.500000000000000000 ) ) ;
#8664=ORIENTED_EDGE ( 'NONE', *, *, #3610, .T. ) ;
#8669=ORIENTED_EDGE ( 'NONE', *, *, #7900, .T. ) ;
#8679=ORIENTED_EDGE ( 'NONE', *, *, #7285, .T. ) ;
#8685=VECTOR ( 'NONE', #9046, 1000.000000000000000 ) ;
#8689=DIRECTION ( 'NONE',  ( -0.000000000000000000, 0.000000000000000000, -1.000000000000000000 ) ) ;
#8696=CARTESIAN_POINT ( 'NONE',  ( 25.00000000000001421, -34.99999999999999289, 7.500000000000000000 ) ) ;
#8706=ORIENTED_EDGE ( 'NONE', *, *, #13764, .F. ) ;
#8707=CARTESIAN_POINT ( 'NONE',  ( -35.00000000000000000, -4.286263797015736496E-15, -4.000000000000000000 ) ) ;
#8708=VERTEX_POINT ( 'NONE', #12696 ) ;
#8710=CARTESIAN_POINT ( 'NONE',  ( -24.99999999999998934, -100.0000000000065938, -5.046127144261280506 ) ) ;
#8713=VERTEX_POINT ( 'NONE', #13776 ) ;
#8715=DIRECTION ( 'NONE',  ( 0.000000000000000000, 0.000000000000000000, 1.000000000000000000 ) ) ;
#8722=DIRECTION ( 'NONE',  ( 0.000000000000000000, 0.000000000000000000, 1.000000000000000000 ) ) ;
#8727=DIRECTION ( 'NONE',  ( 1.000000000000000000, 0.000000000000000000, 0.000000000000000000 ) ) ;
#8732=CARTESIAN_POINT ( 'NONE',  ( -22.00000000000000000, -35.00000000000000000, -7.500000000000000000 ) ) ;
#8733=EDGE_CURVE ( 'NONE', #11307, #11449, #7558, .T. ) ;
#8739=CIRCLE ( 'NONE', #6720, 2.500000000000002220 ) ;
#8741=LINE ( 'NONE', #13044, #1946 ) ;
#8750=EDGE_CURVE ( 'NONE', #1592, #3741, #6670, .T. ) ;
#8757=CARTESIAN_POINT ( 'NONE',  ( -24.99999999999998934, -99.15310334213020838, 4.530792947966844994E-20 ) ) ;
#8761=ORIENTED_EDGE ( 'NONE', *, *, #7894, .F. ) ;
#8766=CARTESIAN_POINT ( 'NONE',  ( -34.99999999999999289, -97.00000000000000000, -7.500000000000000000 ) ) ;
#8775=EDGE_CURVE ( 'NONE', #12409, #11721, #1301, .T. ) ;
#8777=FACE_OUTER_BOUND ( 'NONE', #4769, .T. ) ;
#8780=FACE_OUTER_BOUND ( 'NONE', #10721, .T. ) ;
#8784=FACE_OUTER_BOUND ( 'NONE', #1605, .T. ) ;
#8792=DIRECTION ( 'NONE',  ( 1.000000000000000000, 0.000000000000000000, 0.000000000000000000 ) ) ;
#8794=CARTESIAN_POINT ( 'NONE',  ( 18.54049621773915746, 27.07720798312000809, -7.500000000000000000 ) ) ;
#8796=CARTESIAN_POINT ( 'NONE',  ( 26.79177319725820539, -26.24642857144861807, 4.000000000000000000 ) ) ;
#8799=EDGE_CURVE ( 'NONE', #12162, #6130, #3098, .T. ) ;
#8802=ORIENTED_EDGE ( 'NONE', *, *, #3548, .T. ) ;
#8805=SHAPE_DEFINITION_REPRESENTATION ( #10664, #2342 ) ;
#8811=AXIS2_PLACEMENT_3D ( 'NONE', #11338, #9100, #7976 ) ;
#8818=ORIENTED_EDGE ( 'NONE', *, *, #13603, .T. ) ;
#8826=DIRECTION ( 'NONE',  ( -0.000000000000000000, -0.000000000000000000, -1.000000000000000000 ) ) ;
#8828=EDGE_CURVE ( 'NONE', #12409, #8361, #7686, .T. ) ;
#8830=ADVANCED_FACE ( 'NONE', ( #1053, #5517 ), #11830, .T. ) ;
#8831=ORIENTED_EDGE ( 'NONE', *, *, #133, .T. ) ;
#8847=DIRECTION ( 'NONE',  ( 0.000000000000000000, 0.000000000000000000, -1.000000000000000000 ) ) ;
#8849=CARTESIAN_POINT ( 'NONE',  ( 0.000000000000000000, 40.00000000000000000, 0.000000000000000000 ) ) ;
#8852=ORIENTED_EDGE ( 'NONE', *, *, #12471, .T. ) ;
#8855=CARTESIAN_POINT ( 'NONE',  ( 37.50000000000000711, 4.592425496802575156E-15, 4.000000000000000000 ) ) ;
#8856=VECTOR ( 'NONE', #6063, 1000.000000000000000 ) ;
#8860=CARTESIAN_POINT ( 'NONE',  ( -60.00000000000001421, -4.286263797015736496E-15, 7.500000000000000000 ) ) ;
#8866=DIRECTION ( 'NONE',  ( 1.000000000000000000, 0.000000000000000000, 0.000000000000000000 ) ) ;
#8871=FACE_BOUND ( 'NONE', #8213, .T. ) ;
#8873=DIRECTION ( 'NONE',  ( -1.000000000000000000, 0.000000000000000000, 0.000000000000000000 ) ) ;
#8877=ORIENTED_EDGE ( 'NONE', *, *, #1891, .F. ) ;
#8884=CARTESIAN_POINT ( 'NONE',  ( -26.79177319725820894, -26.24642857144861807, -4.000000000000000000 ) ) ;
#8886=CARTESIAN_POINT ( 'NONE',  ( -35.00000000000000711, -25.00000000000000711, 7.500000000000000000 ) ) ;
#8888=CYLINDRICAL_SURFACE ( 'NONE', #10581, 25.50000000002550138 ) ;
#8894=VERTEX_POINT ( 'NONE', #9732 ) ;
#8900=CARTESIAN_POINT ( 'NONE',  ( 1.653273178848927024E-14, -135.0000000000000000, 0.000000000000000000 ) ) ;
#8903=CARTESIAN_POINT ( 'NONE',  ( 18.78199004159288066, 27.01526789321293265, 6.903011289631059810 ) ) ;
#8909=AXIS2_PLACEMENT_3D ( 'NONE', #3134, #907, #1953 ) ;
#8934=DIRECTION ( 'NONE',  ( 0.000000000000000000, 0.000000000000000000, 1.000000000000000000 ) ) ;
#8945=LINE ( 'NONE', #5496, #9071 ) ;
#8948=CARTESIAN_POINT ( 'NONE',  ( -35.00000000000000000, -35.00000000000000000, 7.500000000000000000 ) ) ;
#8958=AXIS2_PLACEMENT_3D ( 'NONE', #10532, #11456, #939 ) ;
#8960=DIRECTION ( 'NONE',  ( -1.000000000000000000, 0.000000000000000000, 0.000000000000000000 ) ) ;
#8963=DIRECTION ( 'NONE',  ( -1.000000000000000000, 0.000000000000000000, 0.000000000000000000 ) ) ;
#8972=CIRCLE ( 'NONE', #3574, 10.00000000000000178 ) ;
#8983=AXIS2_PLACEMENT_3D ( 'NONE', #8261, #11416, #8197 ) ;
#8984=VERTEX_POINT ( 'NONE', #10982 ) ;
#8987=EDGE_LOOP ( 'NONE', ( #2547, #4049, #9984, #3615 ) ) ;
#8989=CARTESIAN_POINT ( 'NONE',  ( 19.18070798040252356, 20.00000000000000000, -4.000000000000000000 ) ) ;
#9009=CARTESIAN_POINT ( 'NONE',  ( 28.79177319725820183, -26.24642857144861807, -4.000000000000000000 ) ) ;
#9018=DIRECTION ( 'NONE',  ( 0.000000000000000000, 0.000000000000000000, 1.000000000000000000 ) ) ;
#9020=DIRECTION ( 'NONE',  ( 0.000000000000000000, 1.000000000000000000, 0.000000000000000000 ) ) ;
#9025=EDGE_LOOP ( 'NONE', ( #2979, #2052, #12360, #2605 ) ) ;
#9034=VECTOR ( 'NONE', #9941, 1000.000000000000000 ) ;
#9035=LINE ( 'NONE', #4889, #2622 ) ;
#9044=VERTEX_POINT ( 'NONE', #2797 ) ;
#9045=CARTESIAN_POINT ( 'NONE',  ( 25.00000000000001776, -100.0000000000000000, 7.500000000000000000 ) ) ;
#9046=DIRECTION ( 'NONE',  ( -1.224646799147353207E-16, 1.000000000000000000, -0.000000000000000000 ) ) ;
#9057=CIRCLE ( 'NONE', #3441, 20.00000000000000000 ) ;
#9059=CARTESIAN_POINT ( 'NONE',  ( 35.00000000000000000, -4.286263797015736496E-15, 4.000000000000000000 ) ) ;
#9060=LINE ( 'NONE', #8989, #473 ) ;
#9065=CARTESIAN_POINT ( 'NONE',  ( 35.00000000000000000, -4.286263797015736496E-15, 4.000000000000000000 ) ) ;
#9068=AXIS2_PLACEMENT_3D ( 'NONE', #11824, #9392, #5308 ) ;
#9069=CARTESIAN_POINT ( 'NONE',  ( 15.70039857998626864, -16.66659488452782156, -0.6827713257413515757 ) ) ;
#9071=VECTOR ( 'NONE', #13248, 1000.000000000000000 ) ;
#9072=ORIENTED_EDGE ( 'NONE', *, *, #4649, .T. ) ;
#9073=ORIENTED_EDGE ( 'NONE', *, *, #8799, .F. ) ;
#9074=DIRECTION ( 'NONE',  ( -0.000000000000000000, -0.000000000000000000, -1.000000000000000000 ) ) ;
#9082=CIRCLE ( 'NONE', #6833, 35.00000000000000000 ) ;
#9092=DIRECTION ( 'NONE',  ( 0.000000000000000000, -1.000000000000000000, 0.000000000000000000 ) ) ;
#9095=PRODUCT_DEFINITION_FORMATION_WITH_SPECIFIED_SOURCE ( 'ANY', '', #1387, .NOT_KNOWN. ) ;
#9100=DIRECTION ( 'NONE',  ( -0.000000000000000000, -0.000000000000000000, -1.000000000000000000 ) ) ;
#9107=EDGE_CURVE ( 'NONE', #11721, #4007, #12619, .T. ) ;
#9111=EDGE_LOOP ( 'NONE', ( #2361, #2624, #12843, #5769 ) ) ;
#9113=VERTEX_POINT ( 'NONE', #7332 ) ;
#9122=CARTESIAN_POINT ( 'NONE',  ( 18.54049621773915746, -20.00000000000000000, 7.500000000000000000 ) ) ;
#9123=VERTEX_POINT ( 'NONE', #7064 ) ;
#9125=ORIENTED_EDGE ( 'NONE', *, *, #4138, .T. ) ;
#9136=CARTESIAN_POINT ( 'NONE',  ( 37.50000000000000711, 4.592425496802575156E-15, 7.500000000000000000 ) ) ;
#9137=CARTESIAN_POINT ( 'NONE',  ( -15.18222645069203125, 20.00000000000000355, 4.000000000000000000 ) ) ;
#9146=ORIENTED_EDGE ( 'NONE', *, *, #8343, .T. ) ;
#9148=CARTESIAN_POINT ( 'NONE',  ( 23.10070469010960537, -97.98123128958475547, -7.500000000000000000 ) ) ;
#9156=ORIENTED_EDGE ( 'NONE', *, *, #133, .F. ) ;
#9161=VECTOR ( 'NONE', #4965, 1000.000000000000000 ) ;
#9164=CARTESIAN_POINT ( 'NONE',  ( -15.64391473689848233, -16.60099851263468196, -1.372939470208868196 ) ) ;
#9169=CARTESIAN_POINT ( 'NONE',  ( -32.50000000000000000, -3.980102097228898626E-15, 4.000000000000000000 ) ) ;
#9178=ADVANCED_FACE ( 'NONE', ( #9654, #3263 ), #4443, .T. ) ;
#9179=CARTESIAN_POINT ( 'NONE',  ( 35.00000000000000000, 4.286263797015736496E-15, -4.000000000000000000 ) ) ;
#9181=VECTOR ( 'NONE', #12604, 1000.000000000000000 ) ;
#9204=DIRECTION ( 'NONE',  ( -1.224646799147353207E-16, 1.000000000000000000, -0.000000000000000000 ) ) ;
#9212=ORIENTED_EDGE ( 'NONE', *, *, #8153, .T. ) ;
#9221=ORIENTED_EDGE ( 'NONE', *, *, #5771, .F. ) ;
#9227=DIRECTION ( 'NONE',  ( 0.000000000000000000, -0.000000000000000000, 1.000000000000000000 ) ) ;
#9235=ORIENTED_EDGE ( 'NONE', *, *, #4796, .F. ) ;
#9240=CARTESIAN_POINT ( 'NONE',  ( -15.70027825049740500, -16.66645554390144568, -0.3441452025673427118 ) ) ;
#9243=CARTESIAN_POINT ( 'NONE',  ( -21.99999999999999289, -100.0000000000000000, 7.500000000000000000 ) ) ;
#9269=CARTESIAN_POINT ( 'NONE',  ( -15.49340857339600319, -22.63585399314533930, -2.623848604783063365 ) ) ;
#9273=DIRECTION ( 'NONE',  ( 0.000000000000000000, 0.000000000000000000, 1.000000000000000000 ) ) ;
#9274=CARTESIAN_POINT ( 'NONE',  ( 35.00000000000001421, -34.99999999999999289, -7.500000000000000000 ) ) ;
#9299=DIRECTION ( 'NONE',  ( -1.000000000000000000, -1.601283208593975514E-16, 0.000000000000000000 ) ) ;
#9300=ORIENTED_EDGE ( 'NONE', *, *, #11526, .F. ) ;
#9304=CIRCLE ( 'NONE', #6381, 66.24999999999978684 ) ;
#9308=CARTESIAN_POINT ( 'NONE',  ( 15.69972745459287466, -22.78055882083339512, 0.6693078754302104194 ) ) ;
#9311=AXIS2_PLACEMENT_3D ( 'NONE', #9481, #6053, #1971 ) ;
#9315=AXIS2_PLACEMENT_3D ( 'NONE', #3092, #4142, #3944 ) ;
#9332=ORIENTED_EDGE ( 'NONE', *, *, #5466, .F. ) ;
#9334=DIRECTION ( 'NONE',  ( -0.000000000000000000, -0.000000000000000000, -1.000000000000000000 ) ) ;
#9335=EDGE_LOOP ( 'NONE', ( #8818, #7937, #986, #2450 ) ) ;
#9338=AXIS2_PLACEMENT_3D ( 'NONE', #9940, #3541, #10225 ) ;
#9339=ORIENTED_EDGE ( 'NONE', *, *, #8775, .T. ) ;
#9341=ORIENTED_EDGE ( 'NONE', *, *, #12631, .T. ) ;
#9345=LINE ( 'NONE', #11514, #1335 ) ;
#9349=ORIENTED_EDGE ( 'NONE', *, *, #9849, .F. ) ;
#9365=CARTESIAN_POINT ( 'NONE',  ( 25.00000000000002487, -99.43893449056523082, -2.967955073073426764 ) ) ;
#9370=DIRECTION ( 'NONE',  ( -1.000000000000000000, 0.000000000000000000, 0.000000000000000000 ) ) ;
#9375=LINE ( 'NONE', #2717, #9538 ) ;
#9376=DIRECTION ( 'NONE',  ( -1.000000000000000000, -1.224646799147353207E-16, 0.000000000000000000 ) ) ;
#9388=AXIS2_PLACEMENT_3D ( 'NONE', #2889, #450, #1625 ) ;
#9392=DIRECTION ( 'NONE',  ( 0.000000000000000000, 0.000000000000000000, 1.000000000000000000 ) ) ;
#9400=AXIS2_PLACEMENT_3D ( 'NONE', #1653, #5936, #6840 ) ;
#9402=CYLINDRICAL_SURFACE ( 'NONE', #11521, 2.500000000000002220 ) ;
#9405=ORIENTED_EDGE ( 'NONE', *, *, #8343, .F. ) ;
#9411=CARTESIAN_POINT ( 'NONE',  ( -15.36839996672162556, -22.54980054760556385, -3.276782387371333982 ) ) ;
#9417=AXIS2_PLACEMENT_3D ( 'NONE', #2623, #11309, #10125 ) ;
#9420=ORIENTED_EDGE ( 'NONE', *, *, #3896, .F. ) ;
#9424=CIRCLE ( 'NONE', #6277, 2.500000000000002220 ) ;
#9432=FACE_OUTER_BOUND ( 'NONE', #5198, .T. ) ;
#9444=VERTEX_POINT ( 'NONE', #9826 ) ;
#9446=VERTEX_POINT ( 'NONE', #10933 ) ;
#9460=ADVANCED_FACE ( 'NONE', ( #5538 ), #13472, .F. ) ;
#9469=ORIENTED_EDGE ( 'NONE', *, *, #11920, .T. ) ;
#9479=LINE ( 'NONE', #1061, #9585 ) ;
#9480=CARTESIAN_POINT ( 'NONE',  ( -15.65828099947304253, -22.75074427536020494, -1.322318745440853593 ) ) ;
#9481=CARTESIAN_POINT ( 'NONE',  ( -35.00000000000012079, 91.25000000000045475, -4.000000000000000000 ) ) ;
#9495=CARTESIAN_POINT ( 'NONE',  ( 0.000000000000000000, -100.0000000000000000, 15.70031846811053455 ) ) ;
#9497=CIRCLE ( 'NONE', #11043, 66.25000000000044054 ) ;
#9502=CARTESIAN_POINT ( 'NONE',  ( -24.99999999999998934, -100.0000000000000000, 7.500000000000000000 ) ) ;
#9507=AXIS2_PLACEMENT_3D ( 'NONE', #8884, #3536, #8963 ) ;
#9527=EDGE_CURVE ( 'NONE', #12788, #4855, #7512, .T. ) ;
#9530=EDGE_CURVE ( 'NONE', #13109, #6662, #7582, .T. ) ;
#9535=VERTEX_POINT ( 'NONE', #5407 ) ;
#9537=CARTESIAN_POINT ( 'NONE',  ( 1.387778780781445676E-14, -100.0000000000000000, 0.000000000000000000 ) ) ;
#9538=VECTOR ( 'NONE', #1593, 1000.000000000000000 ) ;
#9544=CARTESIAN_POINT ( 'NONE',  ( 35.00000000000000000, 4.286263797015736496E-15, -4.000000000000000000 ) ) ;
#9545=AXIS2_PLACEMENT_3D ( 'NONE', #5124, #6452, #6582 ) ;
#9546=CARTESIAN_POINT ( 'NONE',  ( -15.49491024508755999, -22.63688244086937118, 2.616826951557487568 ) ) ;
#9553=VERTEX_POINT ( 'NONE', #11720 ) ;
#9557=CIRCLE ( 'NONE', #8221, 15.70031846811053455 ) ;
#9561=LINE ( 'NONE', #9495, #896 ) ;
#9564=CYLINDRICAL_SURFACE ( 'NONE', #4949, 1.999999999999998224 ) ;
#9567=DIRECTION ( 'NONE',  ( -0.000000000000000000, 0.000000000000000000, -1.000000000000000000 ) ) ;
#9573=FACE_OUTER_BOUND ( 'NONE', #12918, .T. ) ;
#9584=ORIENTED_EDGE ( 'NONE', *, *, #12631, .F. ) ;
#9585=VECTOR ( 'NONE', #10393, 1000.000000000000000 ) ;
#9604=ORIENTED_EDGE ( 'NONE', *, *, #61, .T. ) ;
#9609=CYLINDRICAL_SURFACE ( 'NONE', #2700, 66.25000000000044054 ) ;
#9610=CARTESIAN_POINT ( 'NONE',  ( -24.99999999999998579, -99.15310334213020838, 0.8520627238941246295 ) ) ;
#9614=EDGE_CURVE ( 'NONE', #5523, #4125, #6256, .T. ) ;
#9618=CIRCLE ( 'NONE', #13486, 69.24999999999975842 ) ;
#9620=EDGE_CURVE ( 'NONE', #7192, #4098, #2903, .T. ) ;
#9625=DIRECTION ( 'NONE',  ( -1.000000000000000000, -1.224646799147353207E-16, 0.000000000000000000 ) ) ;
#9629=DIRECTION ( 'NONE',  ( -1.000000000000000000, 0.000000000000000000, 0.000000000000000000 ) ) ;
#9634=CARTESIAN_POINT ( 'NONE',  ( 13.79311422413708499, -20.00000000000000355, -7.500000000000000000 ) ) ;
#9636=VECTOR ( 'NONE', #1954, 1000.000000000000000 ) ;
#9638=ADVANCED_FACE ( 'NONE', ( #7240 ), #11655, .T. ) ;
#9642=VERTEX_POINT ( 'NONE', #8297 ) ;
#9643=CARTESIAN_POINT ( 'NONE',  ( 22.00000000000000355, -34.99999999999999289, 7.500000000000000000 ) ) ;
#9644=FACE_OUTER_BOUND ( 'NONE', #13289, .T. ) ;
#9654=FACE_OUTER_BOUND ( 'NONE', #11718, .T. ) ;
#9658=ORIENTED_EDGE ( 'NONE', *, *, #13630, .F. ) ;
#9662=CARTESIAN_POINT ( 'NONE',  ( -19.38529118556630237, 26.86594603178323482, 5.082853661574513460 ) ) ;
#9674=DIRECTION ( 'NONE',  ( 1.224646799147353207E-16, -1.000000000000000000, 0.000000000000000000 ) ) ;
#9676=CARTESIAN_POINT ( 'NONE',  ( -60.00000000000001421, 20.00000000000000000, 4.000000000000000000 ) ) ;
#9687=ADVANCED_FACE ( 'NONE', ( #2378 ), #7709, .T. ) ;
#9691=ADVANCED_FACE ( 'NONE', ( #5468 ), #11005, .T. ) ;
#9702=CIRCLE ( 'NONE', #4532, 15.70031846811053455 ) ;
#9705=DIRECTION ( 'NONE',  ( -1.000000000000000000, -1.224646799147353207E-16, 0.000000000000000000 ) ) ;
#9719=CARTESIAN_POINT ( 'NONE',  ( 27.38873514654796537, -24.33759740261776017, 4.000000000000000000 ) ) ;
#9725=ORIENTED_EDGE ( 'NONE', *, *, #4851, .T. ) ;
#9729=AXIS2_PLACEMENT_3D ( 'NONE', #8519, #2072, #8321 ) ;
#9730=CARTESIAN_POINT ( 'NONE',  ( -19.96844336951937748, 26.72776445485856200, 1.294012040295340782 ) ) ;
#9732=CARTESIAN_POINT ( 'NONE',  ( 30.72062512117245703, 25.13835616439070719, -4.000000000000000000 ) ) ;
#9741=DIRECTION ( 'NONE',  ( 1.000000000000000000, 1.224646799147353207E-16, 0.000000000000000000 ) ) ;
#9742=CARTESIAN_POINT ( 'NONE',  ( 22.00000000000002132, -100.0000000000000000, -7.500000000000000000 ) ) ;
#9745=PLANE ( 'NONE',  #3651 ) ;
#9748=AXIS2_PLACEMENT_3D ( 'NONE', #12442, #605, #1640 ) ;
#9755=LINE ( 'NONE', #8766, #4699 ) ;
#9770=DIRECTION ( 'NONE',  ( -0.000000000000000000, -0.000000000000000000, -1.000000000000000000 ) ) ;
#9774=DIRECTION ( 'NONE',  ( 1.000000000000000000, 0.000000000000000000, 0.000000000000000000 ) ) ;
#9775=DIRECTION ( 'NONE',  ( -1.224646799147353207E-16, 1.000000000000000000, -0.000000000000000000 ) ) ;
#9779=ORIENTED_EDGE ( 'NONE', *, *, #4838, .F. ) ;
#9781=CARTESIAN_POINT ( 'NONE',  ( -23.09891356890234348, -97.97864346908494326, -7.500000000000000000 ) ) ;
#9796=ADVANCED_FACE ( 'NONE', ( #165 ), #3724, .F. ) ;
#9800=CARTESIAN_POINT ( 'NONE',  ( 37.50000000000000711, 4.592425496802575156E-15, 7.500000000000000000 ) ) ;
#9801=CARTESIAN_POINT ( 'NONE',  ( 35.00000000000000000, -4.286263797015736496E-15, -4.000000000000000000 ) ) ;
#9803=ORIENTED_EDGE ( 'NONE', *, *, #2929, .F. ) ;
#9806=ORIENTED_EDGE ( 'NONE', *, *, #11266, .F. ) ;
#9817=DIRECTION ( 'NONE',  ( -1.000000000000000000, 0.000000000000000000, 0.000000000000000000 ) ) ;
#9822=DIRECTION ( 'NONE',  ( -1.000000000000000000, 0.000000000000000000, 0.000000000000000000 ) ) ;
#9824=PLANE ( 'NONE',  #6790 ) ;
#9826=CARTESIAN_POINT ( 'NONE',  ( -21.99999999999999289, -97.00000000000000000, -7.500000000000000000 ) ) ;
#9835=ORIENTED_EDGE ( 'NONE', *, *, #8494, .T. ) ;
#9836=CARTESIAN_POINT ( 'NONE',  ( -19.18070798040252356, 20.00000000000000000, 4.000000000000000000 ) ) ;
#9838=ORIENTED_EDGE ( 'NONE', *, *, #6789, .T. ) ;
#9839=CYLINDRICAL_SURFACE ( 'NONE', #4495, 15.70031846811053455 ) ;
#9842=CARTESIAN_POINT ( 'NONE',  ( 1.653273178848927024E-14, -135.0000000000000000, 0.000000000000000000 ) ) ;
#9844=CARTESIAN_POINT ( 'NONE',  ( -37.50000000000000711, -4.286263797015736496E-15, 4.000000000000000000 ) ) ;
#9849=EDGE_CURVE ( 'NONE', #1947, #3433, #8597, .T. ) ;
#9852=EDGE_CURVE ( 'NONE', #3741, #7494, #12218, .T. ) ;
#9855=CIRCLE ( 'NONE', #5367, 25.00000000000000355 ) ;
#9869=EDGE_CURVE ( 'NONE', #6733, #3737, #11297, .T. ) ;
#9871=CARTESIAN_POINT ( 'NONE',  ( 25.00000000000001776, -100.0000000000064801, 5.046127144260958097 ) ) ;
#9873=CYLINDRICAL_SURFACE ( 'NONE', #4994, 25.00000000000000711 ) ;
#9887=FACE_OUTER_BOUND ( 'NONE', #7626, .T. ) ;
#9892=CARTESIAN_POINT ( 'NONE',  ( 35.00000000000000711, -25.00000000000000000, 7.500000000000000000 ) ) ;
#9899=CARTESIAN_POINT ( 'NONE',  ( -26.79177319725820894, -26.24642857144861807, -4.000000000000000000 ) ) ;
#9902=SURFACE_SIDE_STYLE ('',( #2459 ) ) ;
#9906=CARTESIAN_POINT ( 'NONE',  ( 0.000000000000000000, 0.000000000000000000, 0.000000000000000000 ) ) ;
#9911=DIRECTION ( 'NONE',  ( -0.000000000000000000, -0.000000000000000000, -1.000000000000000000 ) ) ;
#9912=LINE ( 'NONE', #11941, #13814 ) ;
#9915=EDGE_LOOP ( 'NONE', ( #10010, #2787, #11177, #5881 ) ) ;
#9918=CYLINDRICAL_SURFACE ( 'NONE', #1912, 10.00000000000000178 ) ;
#9923=CARTESIAN_POINT ( 'NONE',  ( -35.00000000000000000, -20.00000000000000000, -7.500000000000000000 ) ) ;
#9924=FACE_OUTER_BOUND ( 'NONE', #13398, .T. ) ;
#9927=VECTOR ( 'NONE', #2103, 1000.000000000000000 ) ;
#9931=VERTEX_POINT ( 'NONE', #2879 ) ;
#9939=DIRECTION ( 'NONE',  ( -0.000000000000000000, -0.000000000000000000, -1.000000000000000000 ) ) ;
#9940=CARTESIAN_POINT ( 'NONE',  ( 35.00000000000000000, 4.286263797015736496E-15, 7.500000000000000000 ) ) ;
#9941=DIRECTION ( 'NONE',  ( 0.000000000000000000, -1.000000000000000000, 0.000000000000000000 ) ) ;
#9946=ADVANCED_FACE ( 'NONE', ( #6311 ), #5235, .F. ) ;
#9948=ADVANCED_FACE ( 'NONE', ( #7154 ), #1755, .F. ) ;
#9957=DIRECTION ( 'NONE',  ( 1.000000000000000000, 0.000000000000000000, 0.000000000000000000 ) ) ;
#9962=ORIENTED_EDGE ( 'NONE', *, *, #4796, .T. ) ;
#9973=DIRECTION ( 'NONE',  ( -1.000000000000000000, 0.000000000000000000, 0.000000000000000000 ) ) ;
#9977=AXIS2_PLACEMENT_3D ( 'NONE', #6481, #3311, #1162 ) ;
#9984=ORIENTED_EDGE ( 'NONE', *, *, #7375, .T. ) ;
#9985=ORIENTED_EDGE ( 'NONE', *, *, #8570, .T. ) ;
#9986=CARTESIAN_POINT ( 'NONE',  ( -22.00000000000000000, -2.694222958124176809E-15, 0.000000000000000000 ) ) ;
#9987=DIRECTION ( 'NONE',  ( -1.224646799147353207E-16, -1.499759782661857608E-32, 1.000000000000000000 ) ) ;
#9993=DIRECTION ( 'NONE',  ( -0.000000000000000000, -0.000000000000000000, -1.000000000000000000 ) ) ;
#10002=CARTESIAN_POINT ( 'NONE',  ( -21.99999999999999289, -100.0000000000000000, -7.500000000000000000 ) ) ;
#10009=CARTESIAN_POINT ( 'NONE',  ( 34.99999999999999289, 25.00000000000002132, 7.500000000000000000 ) ) ;
#10010=ORIENTED_EDGE ( 'NONE', *, *, #12641, .T. ) ;
#10020=ORIENTED_EDGE ( 'NONE', *, *, #1895, .F. ) ;
#10023=CARTESIAN_POINT ( 'NONE',  ( 1.187907395172932673E-14, -97.00000000000000000, 0.000000000000000000 ) ) ;
#10027=ADVANCED_FACE ( 'NONE', ( #985 ), #9402, .F. ) ;
#10035=AXIS2_PLACEMENT_3D ( 'NONE', #13305, #3581, #11303 ) ;
#10037=EDGE_LOOP ( 'NONE', ( #557, #107, #12420, #11698 ) ) ;
#10048=CARTESIAN_POINT ( 'NONE',  ( 15.61050411040038099, -16.56206589787452188, 1.710375830838840816 ) ) ;
#10049=ORIENTED_EDGE ( 'NONE', *, *, #10607, .T. ) ;
#10052=CARTESIAN_POINT ( 'NONE',  ( -35.00000000000000000, -4.286263797015736496E-15, -7.500000000000000000 ) ) ;
#10063=PLANE ( 'NONE',  #3337 ) ;
#10064=DIRECTION ( 'NONE',  ( 1.000000000000000000, 0.000000000000000000, -0.000000000000000000 ) ) ;
#10072=ORIENTED_EDGE ( 'NONE', *, *, #7706, .T. ) ;
#10073=LINE ( 'NONE', #6909, #12078 ) ;
#10078=VERTEX_POINT ( 'NONE', #8732 ) ;
#10083=CIRCLE ( 'NONE', #4925, 25.50000000002550138 ) ;
#10087=CARTESIAN_POINT ( 'NONE',  ( 26.79177319725820539, -26.24642857144861807, -4.000000000000000000 ) ) ;
#10095=ORIENTED_EDGE ( 'NONE', *, *, #7285, .F. ) ;
#10100=DIRECTION ( 'NONE',  ( -0.000000000000000000, -0.000000000000000000, 1.000000000000000000 ) ) ;
#10117=PLANE ( 'NONE',  #9388 ) ;
#10122=DIRECTION ( 'NONE',  ( -1.000000000000000000, -1.224646799147353207E-16, 0.000000000000000000 ) ) ;
#10125=DIRECTION ( 'NONE',  ( 1.000000000000000000, 0.000000000000000000, 0.000000000000000000 ) ) ;
#10127=STYLED_ITEM ( 'NONE', ( #3549 ), #3056 ) ;
#10129=LINE ( 'NONE', #5997, #13235 ) ;
#10140=EDGE_CURVE ( 'NONE', #8984, #470, #2505, .T. ) ;
#10145=CARTESIAN_POINT ( 'NONE',  ( -15.18222645069203125, -100.0000000000000000, 4.000000000000000000 ) ) ;
#10159=CARTESIAN_POINT ( 'NONE',  ( -31.93204061526059334, -135.0000000000000000, 0.000000000000000000 ) ) ;
#10166=ORIENTED_EDGE ( 'NONE', *, *, #7138, .F. ) ;
#10170=CARTESIAN_POINT ( 'NONE',  ( 19.51309799441515835, 26.83545189264578212, 4.432601239563248363 ) ) ;
#10174=ORIENTED_EDGE ( 'NONE', *, *, #7196, .T. ) ;
#10183=CARTESIAN_POINT ( 'NONE',  ( 35.00000000000000711, -25.00000000000000000, 7.500000000000000000 ) ) ;
#10191=ORIENTED_EDGE ( 'NONE', *, *, #5847, .T. ) ;
#10200=ORIENTED_EDGE ( 'NONE', *, *, #11155, .T. ) ;
#10201=ORIENTED_EDGE ( 'NONE', *, *, #10970, .F. ) ;
#10208=CARTESIAN_POINT ( 'NONE',  ( 0.000000000000000000, 20.00000000000000355, 0.000000000000000000 ) ) ;
#10210=EDGE_CURVE ( 'NONE', #6099, #10920, #5242, .T. ) ;
#10211=EDGE_CURVE ( 'NONE', #2392, #8894, #5683, .T. ) ;
#10218=ADVANCED_FACE ( 'NONE', ( #2644 ), #6156, .F. ) ;
#10225=DIRECTION ( 'NONE',  ( -1.000000000000000000, 0.000000000000000000, 0.000000000000000000 ) ) ;
#10226=LINE ( 'NONE', #8049, #7232 ) ;
#10227=PRODUCT_DEFINITION_CONTEXT ( 'detailed design', #10837, 'design' ) ;
#10229=ADVANCED_FACE ( 'NONE', ( #827 ), #12541, .T. ) ;
#10232=EDGE_CURVE ( 'NONE', #6733, #8612, #9057, .T. ) ;
#10236=FACE_OUTER_BOUND ( 'NONE', #3845, .T. ) ;
#10237=CARTESIAN_POINT ( 'NONE',  ( 19.99988111993866724, 26.72048013816596779, -0.6453928856983822682 ) ) ;
#10241=VERTEX_POINT ( 'NONE', #2922 ) ;
#10245=CARTESIAN_POINT ( 'NONE',  ( -25.00000000000000000, -35.00000000000000000, -7.500000000000000000 ) ) ;
#10250=DIRECTION ( 'NONE',  ( 1.000000000000000000, 1.601283208593975514E-16, -0.000000000000000000 ) ) ;
#10253=CYLINDRICAL_SURFACE ( 'NONE', #3716, 15.70031846811053455 ) ;
#10255=CARTESIAN_POINT ( 'NONE',  ( 15.64391473689848233, -16.60099851263468196, 1.372939470208868196 ) ) ;
#10258=VERTEX_POINT ( 'NONE', #1594 ) ;
#10262=VECTOR ( 'NONE', #1192, 1000.000000000000000 ) ;
#10273=AXIS2_PLACEMENT_3D ( 'NONE', #9801, #10642, #208 ) ;
#10277=AXIS2_PLACEMENT_3D ( 'NONE', #2385, #171, #234 ) ;
#10280=ORIENTED_EDGE ( 'NONE', *, *, #9614, .T. ) ;
#10286=CARTESIAN_POINT ( 'NONE',  ( -15.34998809918498353, -16.25417180422370933, 3.363251165709652213 ) ) ;
#10300=ADVANCED_FACE ( 'NONE', ( #626 ), #6995, .F. ) ;
#10303=EDGE_CURVE ( 'NONE', #8708, #5686, #2260, .T. ) ;
#10310=PLANE ( 'NONE',  #8423 ) ;
#10314=VERTEX_POINT ( 'NONE', #10618 ) ;
#10325=CARTESIAN_POINT ( 'NONE',  ( -24.99999999999998934, -100.0000000000000000, 7.500000000000000000 ) ) ;
#10337=AXIS2_PLACEMENT_3D ( 'NONE', #7219, #9334, #916 ) ;
#10344=CARTESIAN_POINT ( 'NONE',  ( 2.449293598294706513E-15, 40.00000000000000000, -20.00000000000000000 ) ) ;
#10346=CARTESIAN_POINT ( 'NONE',  ( 31.93204061526061466, -132.0000000000000000, 3.910547132972217398E-15 ) ) ;
#10357=DIRECTION ( 'NONE',  ( 1.000000000000000000, 0.000000000000000000, 0.000000000000000000 ) ) ;
#10361=LINE ( 'NONE', #9243, #10663 ) ;
#10365=EDGE_CURVE ( 'NONE', #12788, #11308, #10616, .T. ) ;
#10367=PLANE ( 'NONE',  #8983 ) ;
#10382=EDGE_CURVE ( 'NONE', #8229, #10692, #3226, .T. ) ;
#10385=ADVANCED_FACE ( 'NONE', ( #9644 ), #8587, .T. ) ;
#10393=DIRECTION ( 'NONE',  ( 1.000000000000000000, -0.000000000000000000, -0.000000000000000000 ) ) ;
#10399=ORIENTED_EDGE ( 'NONE', *, *, #12957, .F. ) ;
#10413=VECTOR ( 'NONE', #1263, 1000.000000000000000 ) ;
#10424=CARTESIAN_POINT ( 'NONE',  ( -15.61050411040038099, -16.56206589787452188, -1.710375830838840816 ) ) ;
#10434=EDGE_LOOP ( 'NONE', ( #3397, #5255, #8239, #9420, #3829, #3164, #6618, #202 ) ) ;
#10442=CARTESIAN_POINT ( 'NONE',  ( 15.18222645069203125, -100.0000000000000000, 4.000000000000000000 ) ) ;
#10445=AXIS2_PLACEMENT_3D ( 'NONE', #333, #13030, #8873 ) ;
#10449=DIRECTION ( 'NONE',  ( -0.000000000000000000, -0.000000000000000000, -1.000000000000000000 ) ) ;
#10459=CARTESIAN_POINT ( 'NONE',  ( -14.85082311557358103, -22.21562007816737960, 5.135570635274604889 ) ) ;
#10464=VERTEX_POINT ( 'NONE', #2004 ) ;
#10473=CARTESIAN_POINT ( 'NONE',  ( 26.79177319725820539, -26.24642857144861807, -4.000000000000000000 ) ) ;
#10480=CARTESIAN_POINT ( 'NONE',  ( -35.00000000000000000, -4.286263797015736496E-15, -4.000000000000000000 ) ) ;
#10484=ORIENTED_EDGE ( 'NONE', *, *, #11502, .F. ) ;
#10485=DIRECTION ( 'NONE',  ( 0.000000000000000000, 0.000000000000000000, 1.000000000000000000 ) ) ;
#10486=CARTESIAN_POINT ( 'NONE',  ( 1.187907395172932673E-14, -97.00000000000000000, 0.000000000000000000 ) ) ;
#10488=CARTESIAN_POINT ( 'NONE',  ( 13.79311422413708499, -21.62638421600850691, 7.500000000000000000 ) ) ;
#10499=ORIENTED_EDGE ( 'NONE', *, *, #2985, .T. ) ;
#10501=CARTESIAN_POINT ( 'NONE',  ( 31.93204061526062176, -135.0000000000000000, 3.910547132972218187E-15 ) ) ;
#10505=CARTESIAN_POINT ( 'NONE',  ( 35.00000000000000000, 4.286263797015736496E-15, -7.500000000000000000 ) ) ;
#10506=ORIENTED_EDGE ( 'NONE', *, *, #12828, .T. ) ;
#10515=EDGE_LOOP ( 'NONE', ( #7748, #4781, #7902, #2549, #9332, #12444, #9838, #5315 ) ) ;
#10516=CARTESIAN_POINT ( 'NONE',  ( 25.00000000000001776, -100.0000000000064801, 5.046127144260958097 ) ) ;
#10518=CARTESIAN_POINT ( 'NONE',  ( 0.000000000000000000, 0.000000000000000000, 0.000000000000000000 ) ) ;
#10519=CARTESIAN_POINT ( 'NONE',  ( -14.88155114952948921, -22.23162151614122450, -5.171026666816163520 ) ) ;
#10529=ORIENTED_EDGE ( 'NONE', *, *, #6701, .F. ) ;
#10532=CARTESIAN_POINT ( 'NONE',  ( -35.00000000000000000, -4.286263797015736496E-15, 7.500000000000000000 ) ) ;
#10541=CARTESIAN_POINT ( 'NONE',  ( 28.15981099771517648, -27.70535714287384721, 4.000000000000000000 ) ) ;
#10544=VECTOR ( 'NONE', #8847, 1000.000000000000000 ) ;
#10546=AXIS2_PLACEMENT_3D ( 'NONE', #11491, #1881, #6169 ) ;
#10548=LINE ( 'NONE', #1018, #13281 ) ;
#10558=DIRECTION ( 'NONE',  ( -1.224646799147353207E-16, 1.000000000000000000, -0.000000000000000000 ) ) ;
#10562=CARTESIAN_POINT ( 'NONE',  ( 15.18222645069203303, -16.04698886238941924, 4.000000000000000000 ) ) ;
#10581=AXIS2_PLACEMENT_3D ( 'NONE', #2219, #4527, #5515 ) ;
#10582=EDGE_CURVE ( 'NONE', #618, #8349, #8945, .T. ) ;
#10584=ORIENTED_EDGE ( 'NONE', *, *, #5847, .F. ) ;
#10589=CARTESIAN_POINT ( 'NONE',  ( -15.70089697932619899, -22.78139155752743861, 0.6412871628180817352 ) ) ;
#10590=CARTESIAN_POINT ( 'NONE',  ( -24.99999999999998224, -99.22499053259343782, 1.700537903188983346 ) ) ;
#10607=EDGE_CURVE ( 'NONE', #9642, #2556, #5766, .T. ) ;
#10608=CARTESIAN_POINT ( 'NONE',  ( 25.00000000000001776, -100.0000000000000000, -5.046127144242417373 ) ) ;
#10610=VECTOR ( 'NONE', #2675, 1000.000000000000000 ) ;
#10616=CIRCLE ( 'NONE', #9729, 25.50418395392908977 ) ;
#10618=CARTESIAN_POINT ( 'NONE',  ( -30.72062512117240018, 25.13835616439069653, 4.000000000000000000 ) ) ;
#10619=CARTESIAN_POINT ( 'NONE',  ( 13.79311422413708499, -21.62638421600850691, -7.500000000000000000 ) ) ;
#10624=EDGE_CURVE ( 'NONE', #5941, #11307, #12664, .T. ) ;
#10628=EDGE_CURVE ( 'NONE', #6696, #7751, #5698, .T. ) ;
#10633=ORIENTED_EDGE ( 'NONE', *, *, #5943, .F. ) ;
#10636=DIRECTION ( 'NONE',  ( -0.000000000000000000, -0.000000000000000000, -1.000000000000000000 ) ) ;
#10638=( GEOMETRIC_REPRESENTATION_CONTEXT ( 3 ) GLOBAL_UNCERTAINTY_ASSIGNED_CONTEXT ( ( #7832 ) ) GLOBAL_UNIT_ASSIGNED_CONTEXT ( ( #6812, #1332, #6595 ) ) REPRESENTATION_CONTEXT ( 'NONE', 'WORKASPACE' ) );
#10641=( NAMED_UNIT ( * ) SI_UNIT ( $, .STERADIAN. ) SOLID_ANGLE_UNIT ( ) );
#10642=DIRECTION ( 'NONE',  ( 0.000000000000000000, 0.000000000000000000, 1.000000000000000000 ) ) ;
#10654=DIRECTION ( 'NONE',  ( -1.000000000000000000, 0.000000000000000000, 0.000000000000000000 ) ) ;
#10662=EDGE_LOOP ( 'NONE', ( #8831, #5965 ) ) ;
#10663=VECTOR ( 'NONE', #5164, 1000.000000000000000 ) ;
#10664=PRODUCT_DEFINITION_SHAPE ( 'NONE', 'NONE',  #3939 ) ;
#10674=CARTESIAN_POINT ( 'NONE',  ( 25.00000000000001776, -100.0000000000000000, 7.500000000000000000 ) ) ;
#10683=CARTESIAN_POINT ( 'NONE',  ( -35.00000000000000000, -4.286263797015736496E-15, 7.500000000000000000 ) ) ;
#10685=DIRECTION ( 'NONE',  ( 1.000000000000000000, -0.000000000000000000, -0.000000000000000000 ) ) ;
#10692=VERTEX_POINT ( 'NONE', #1502 ) ;
#10694=ADVANCED_FACE ( 'NONE', ( #3956 ), #5783, .F. ) ;
#10695=VERTEX_POINT ( 'NONE', #2837 ) ;
#10709=ORIENTED_EDGE ( 'NONE', *, *, #7631, .T. ) ;
#10719=ORIENTED_EDGE ( 'NONE', *, *, #3334, .T. ) ;
#10721=EDGE_LOOP ( 'NONE', ( #463, #11518, #13165, #5631 ) ) ;
#10743=CARTESIAN_POINT ( 'NONE',  ( 0.000000000000000000, -20.00000000000000355, 0.000000000000000000 ) ) ;
#10772=EDGE_CURVE ( 'NONE', #11806, #4480, #9082, .T. ) ;
#10773=CARTESIAN_POINT ( 'NONE',  ( -35.00000000000000000, -20.00000000000000000, -7.500000000000000000 ) ) ;
#10787=ORIENTED_EDGE ( 'NONE', *, *, #2870, .F. ) ;
#10796=CARTESIAN_POINT ( 'NONE',  ( 1.387778780781445676E-14, -135.0000000000000000, 0.000000000000000000 ) ) ;
#10798=DIRECTION ( 'NONE',  ( 0.000000000000000000, 0.000000000000000000, 1.000000000000000000 ) ) ;
#10803=VECTOR ( 'NONE', #13377, 1000.000000000000000 ) ;
#10810=DIRECTION ( 'NONE',  ( 0.000000000000000000, -0.000000000000000000, 1.000000000000000000 ) ) ;
#10817=AXIS2_PLACEMENT_3D ( 'NONE', #4744, #11193, #2977 ) ;
#10826=VECTOR ( 'NONE', #2095, 1000.000000000000000 ) ;
#10829=ORIENTED_EDGE ( 'NONE', *, *, #1729, .T. ) ;
#10836=ORIENTED_EDGE ( 'NONE', *, *, #5567, .F. ) ;
#10837=APPLICATION_CONTEXT ( 'automotive_design' ) ;
#10846=LINE ( 'NONE', #9742, #10262 ) ;
#10864=CARTESIAN_POINT ( 'NONE',  ( 1.387778780781445676E-14, -100.0000000000000000, 0.000000000000000000 ) ) ;
#10874=ORIENTED_EDGE ( 'NONE', *, *, #269, .F. ) ;
#10881=ORIENTED_EDGE ( 'NONE', *, *, #13332, .F. ) ;
#10884=AXIS2_PLACEMENT_3D ( 'NONE', #11951, #260, #6353 ) ;
#10891=CYLINDRICAL_SURFACE ( 'NONE', #4996, 2.500000000000002220 ) ;
#10901=VECTOR ( 'NONE', #13857, 1000.000000000000000 ) ;
#10902=CARTESIAN_POINT ( 'NONE',  ( 25.00000000000001776, -99.15310334213020838, 0.4257687054510573832 ) ) ;
#10915=CIRCLE ( 'NONE', #7342, 25.50000000002550138 ) ;
#10920=VERTEX_POINT ( 'NONE', #5155 ) ;
#10926=AXIS2_PLACEMENT_3D ( 'NONE', #8386, #3058, #4169 ) ;
#10931=DIRECTION ( 'NONE',  ( 0.000000000000000000, 0.000000000000000000, 1.000000000000000000 ) ) ;
#10933=CARTESIAN_POINT ( 'NONE',  ( 25.00000000000001421, -34.99999999999999289, -7.500000000000000000 ) ) ;
#10943=VERTEX_POINT ( 'NONE', #13752 ) ;
#10945=ORIENTED_EDGE ( 'NONE', *, *, #13603, .F. ) ;
#10949=ORIENTED_EDGE ( 'NONE', *, *, #1465, .F. ) ;
#10953=CARTESIAN_POINT ( 'NONE',  ( -23.75056915604791641, -98.97863401284405427, -7.500000000000000000 ) ) ;
#10970=EDGE_CURVE ( 'NONE', #12412, #470, #13370, .T. ) ;
#10971=EDGE_CURVE ( 'NONE', #10943, #9931, #113, .T. ) ;
#10974=CIRCLE ( 'NONE', #4725, 15.70031846811053455 ) ;
#10982=CARTESIAN_POINT ( 'NONE',  ( 34.99999999999999289, 25.00000000000002132, 7.500000000000000000 ) ) ;
#10986=EDGE_CURVE ( 'NONE', #6682, #7192, #9912, .T. ) ;
#10989=ORIENTED_EDGE ( 'NONE', *, *, #8245, .F. ) ;
#10992=CARTESIAN_POINT ( 'NONE',  ( 35.00000000000000000, -4.286263797015736496E-15, -4.000000000000000000 ) ) ;
#10996=LINE ( 'NONE', #5679, #12855 ) ;
#11001=ORIENTED_EDGE ( 'NONE', *, *, #13689, .F. ) ;
#11005=CYLINDRICAL_SURFACE ( 'NONE', #2001, 2.000000000000001776 ) ;
#11016=CYLINDRICAL_SURFACE ( 'NONE', #13383, 31.93204061526060045 ) ;
#11017=DIRECTION ( 'NONE',  ( -0.000000000000000000, -0.000000000000000000, -1.000000000000000000 ) ) ;
#11024=CARTESIAN_POINT ( 'NONE',  ( -24.99999999999998934, -99.29838587104467251, -2.138129719433996545 ) ) ;
#11030=DIRECTION ( 'NONE',  ( -0.000000000000000000, -1.000000000000000000, -0.000000000000000000 ) ) ;
#11043=AXIS2_PLACEMENT_3D ( 'NONE', #123, #5560, #5425 ) ;
#11047=EDGE_LOOP ( 'NONE', ( #8706, #11139, #2526, #2894, #12625, #11574, #10020, #7225, #9073, #1288, #5646, #3399 ) ) ;
#11062=ORIENTED_EDGE ( 'NONE', *, *, #11901, .F. ) ;
#11064=EDGE_CURVE ( 'NONE', #2246, #6588, #7930, .T. ) ;
#11068=ORIENTED_EDGE ( 'NONE', *, *, #7758, .F. ) ;
#11093=EDGE_CURVE ( 'NONE', #4208, #5686, #1916, .T. ) ;
#11096=DIRECTION ( 'NONE',  ( 1.000000000000000000, 0.000000000000000000, 0.000000000000000000 ) ) ;
#11099=CIRCLE ( 'NONE', #2131, 21.99999999999999289 ) ;
#11103=CYLINDRICAL_SURFACE ( 'NONE', #4962, 15.00000000000000000 ) ;
#11137=DIRECTION ( 'NONE',  ( 1.000000000000000000, 0.000000000000000000, 0.000000000000000000 ) ) ;
#11139=ORIENTED_EDGE ( 'NONE', *, *, #719, .F. ) ;
#11141=ADVANCED_FACE ( 'NONE', ( #8784 ), #13018, .T. ) ;
#11148=DIRECTION ( 'NONE',  ( 1.000000000000000000, -0.000000000000000000, -0.000000000000000000 ) ) ;
#11150=CARTESIAN_POINT ( 'NONE',  ( 18.99432778721693893, 26.96223687785628442, 6.295342420724995058 ) ) ;
#11155=EDGE_CURVE ( 'NONE', #8094, #5991, #12445, .T. ) ;
#11160=CIRCLE ( 'NONE', #10035, 2.500000000000002220 ) ;
#11162=ORIENTED_EDGE ( 'NONE', *, *, #11901, .T. ) ;
#11169=CARTESIAN_POINT ( 'NONE',  ( 15.65588872828332612, -16.61546069029112260, -1.359866191199148089 ) ) ;
#11170=CARTESIAN_POINT ( 'NONE',  ( -19.18070798040252711, 20.00000000000000000, -4.000000000000000000 ) ) ;
#11177=ORIENTED_EDGE ( 'NONE', *, *, #10628, .F. ) ;
#11180=EDGE_CURVE ( 'NONE', #8229, #6758, #7880, .T. ) ;
#11184=ORIENTED_EDGE ( 'NONE', *, *, #9527, .T. ) ;
#11185=DIRECTION ( 'NONE',  ( 0.000000000000000000, -0.000000000000000000, -1.000000000000000000 ) ) ;
#11193=DIRECTION ( 'NONE',  ( -0.000000000000000000, -0.000000000000000000, -1.000000000000000000 ) ) ;
#11199=AXIS2_PLACEMENT_3D ( 'NONE', #6546, #6675, #4572 ) ;
#11212=ORIENTED_EDGE ( 'NONE', *, *, #3854, .F. ) ;
#11221=LINE ( 'NONE', #13507, #18 ) ;
#11226=VERTEX_POINT ( 'NONE', #9009 ) ;
#11229=ORIENTED_EDGE ( 'NONE', *, *, #10382, .T. ) ;
#11237=CIRCLE ( 'NONE', #5626, 66.24999999999978684 ) ;
#11258=LINE ( 'NONE', #12593, #7065 ) ;
#11260=CARTESIAN_POINT ( 'NONE',  ( -35.00000000000000000, 25.00000000000000000, 7.500000000000000000 ) ) ;
#11262=DIRECTION ( 'NONE',  ( 1.000000000000000000, 0.000000000000000000, 0.000000000000000000 ) ) ;
#11266=EDGE_CURVE ( 'NONE', #3214, #5941, #7038, .T. ) ;
#11272=CARTESIAN_POINT ( 'NONE',  ( 35.00000000000000000, -4.286263797015736496E-15, -4.000000000000000000 ) ) ;
#11277=DIRECTION ( 'NONE',  ( -1.601283208593975514E-16, 1.000000000000000000, -0.000000000000000000 ) ) ;
#11284=AXIS2_PLACEMENT_3D ( 'NONE', #8849, #1218, #13157 ) ;
#11297=LINE ( 'NONE', #4782, #10610 ) ;
#11302=DIRECTION ( 'NONE',  ( 1.000000000000000000, 0.000000000000000000, 0.000000000000000000 ) ) ;
#11303=DIRECTION ( 'NONE',  ( -1.000000000000000000, 0.000000000000000000, 0.000000000000000000 ) ) ;
#11307=VERTEX_POINT ( 'NONE', #5779 ) ;
#11308=VERTEX_POINT ( 'NONE', #465 ) ;
#11309=DIRECTION ( 'NONE',  ( -0.000000000000000000, -0.000000000000000000, -1.000000000000000000 ) ) ;
#11314=DIRECTION ( 'NONE',  ( -1.000000000000000000, 0.000000000000000000, 0.000000000000000000 ) ) ;
#11319=ADVANCED_FACE ( 'NONE', ( #13229 ), #11016, .F. ) ;
#11328=ADVANCED_FACE ( 'NONE', ( #2542 ), #2684, .T. ) ;
#11338=CARTESIAN_POINT ( 'NONE',  ( -35.00000000000000000, -4.286263797015736496E-15, 7.500000000000000000 ) ) ;
#11346=EDGE_LOOP ( 'NONE', ( #4549, #4765, #3917, #9962, #12977, #1043, #5127, #340, #2498, #10191, #13071, #2285 ) ) ;
#11348=FACE_OUTER_BOUND ( 'NONE', #4784, .T. ) ;
#11362=ORIENTED_EDGE ( 'NONE', *, *, #792, .T. ) ;
#11385=CARTESIAN_POINT ( 'NONE',  ( -24.99999999999998934, -100.0000000000000000, 7.500000000000000000 ) ) ;
#11388=CIRCLE ( 'NONE', #5546, 25.50000000002550138 ) ;
#11389=DIRECTION ( 'NONE',  ( -0.000000000000000000, -1.000000000000000000, -0.000000000000000000 ) ) ;
#11390=LINE ( 'NONE', #10002, #2996 ) ;
#11399=CARTESIAN_POINT ( 'NONE',  ( 0.000000000000000000, -20.00000000000000000, 0.000000000000000000 ) ) ;
#11412=ADVANCED_BREP_SHAPE_REPRESENTATION ( '', ( #3056, #8193 ), #12229 ) ;
#11416=DIRECTION ( 'NONE',  ( -1.000000000000000000, -5.337610695313252124E-17, 0.000000000000000000 ) ) ;
#11423=DIRECTION ( 'NONE',  ( 0.000000000000000000, 0.000000000000000000, 1.000000000000000000 ) ) ;
#11427=ORIENTED_EDGE ( 'NONE', *, *, #4312, .T. ) ;
#11430=VERTEX_POINT ( 'NONE', #3504 ) ;
#11435=EDGE_LOOP ( 'NONE', ( #4953, #4064, #7487, #2847 ) ) ;
#11449=VERTEX_POINT ( 'NONE', #4074 ) ;
#11453=EDGE_LOOP ( 'NONE', ( #767, #9604, #13446, #3771, #13781, #2518, #7141, #7568 ) ) ;
#11456=DIRECTION ( 'NONE',  ( 0.000000000000000000, 0.000000000000000000, 1.000000000000000000 ) ) ;
#11461=CARTESIAN_POINT ( 'NONE',  ( -35.00000000000000000, -4.286263797015736496E-15, 4.000000000000000000 ) ) ;
#11465=VECTOR ( 'NONE', #345, 1000.000000000000000 ) ;
#11471=EDGE_CURVE ( 'NONE', #5663, #1107, #1698, .T. ) ;
#11473=ORIENTED_EDGE ( 'NONE', *, *, #7196, .F. ) ;
#11475=CARTESIAN_POINT ( 'NONE',  ( -15.65588872828332612, -16.61546069029112260, 1.359866191199148089 ) ) ;
#11476=( GEOMETRIC_REPRESENTATION_CONTEXT ( 3 ) GLOBAL_UNCERTAINTY_ASSIGNED_CONTEXT ( ( #4609 ) ) GLOBAL_UNIT_ASSIGNED_CONTEXT ( ( #4684, #12761, #10641 ) ) REPRESENTATION_CONTEXT ( 'NONE', 'WORKASPACE' ) );
#11477=CARTESIAN_POINT ( 'NONE',  ( 15.66041902283167175, -22.75225252538438880, -1.300500990791221501 ) ) ;
#11483=VERTEX_POINT ( 'NONE', #13528 ) ;
#11484=EDGE_CURVE ( 'NONE', #10464, #1545, #3039, .T. ) ;
#11491=CARTESIAN_POINT ( 'NONE',  ( 1.224646799147353217E-14, -100.0000000000000000, 0.000000000000000000 ) ) ;
#11493=CARTESIAN_POINT ( 'NONE',  ( 32.50000000000000000, 4.286263797015736496E-15, 7.500000000000000000 ) ) ;
#11494=LINE ( 'NONE', #10442, #9636 ) ;
#11502=EDGE_CURVE ( 'NONE', #8273, #6457, #6253, .T. ) ;
#11503=EDGE_LOOP ( 'NONE', ( #4695, #536, #5634, #10529 ) ) ;
#11507=ORIENTED_EDGE ( 'NONE', *, *, #3269, .T. ) ;
#11510=AXIS2_PLACEMENT_3D ( 'NONE', #1926, #3964, #948 ) ;
#11511=ADVANCED_FACE ( 'NONE', ( #8151, #8217 ), #10253, .F. ) ;
#11512=CARTESIAN_POINT ( 'NONE',  ( -32.50000000000000000, -3.980102097228898626E-15, 7.500000000000000000 ) ) ;
#11513=LINE ( 'NONE', #1969, #737 ) ;
#11514=CARTESIAN_POINT ( 'NONE',  ( 25.00000000000000711, -34.99999999999999289, -7.500000000000000000 ) ) ;
#11518=ORIENTED_EDGE ( 'NONE', *, *, #7372, .F. ) ;
#11521=AXIS2_PLACEMENT_3D ( 'NONE', #12640, #10449, #7292 ) ;
#11526=EDGE_CURVE ( 'NONE', #3127, #11226, #8198, .T. ) ;
#11532=CARTESIAN_POINT ( 'NONE',  ( 25.00000000000000711, -99.22499053259345203, -1.700537903189176525 ) ) ;
#11536=ORIENTED_EDGE ( 'NONE', *, *, #8544, .F. ) ;
#11538=CARTESIAN_POINT ( 'NONE',  ( 25.00000000000000711, -34.99999999999999289, 7.500000000000000000 ) ) ;
#11543=DIRECTION ( 'NONE',  ( -0.000000000000000000, -0.000000000000000000, -1.000000000000000000 ) ) ;
#11554=ORIENTED_EDGE ( 'NONE', *, *, #979, .T. ) ;
#11558=EDGE_LOOP ( 'NONE', ( #3415, #5153, #1305, #4882 ) ) ;
#11561=CYLINDRICAL_SURFACE ( 'NONE', #201, 1.999999999999998224 ) ;
#11574=ORIENTED_EDGE ( 'NONE', *, *, #8828, .T. ) ;
#11587=ORIENTED_EDGE ( 'NONE', *, *, #5225, .F. ) ;
#11590=ADVANCED_FACE ( 'NONE', ( #3942 ), #2891, .F. ) ;
#11603=CARTESIAN_POINT ( 'NONE',  ( -30.72062512117230426, 25.13835616439067877, 0.000000000000000000 ) ) ;
#11621=CARTESIAN_POINT ( 'NONE',  ( -21.99999999999999289, -97.00000000000000000, 7.500000000000000000 ) ) ;
#11630=AXIS2_PLACEMENT_3D ( 'NONE', #8948, #13253, #12453 ) ;
#11636=EDGE_LOOP ( 'NONE', ( #9469, #2666, #10399, #2092, #11657, #6940, #2448, #7305 ) ) ;
#11638=ORIENTED_EDGE ( 'NONE', *, *, #2144, .F. ) ;
#11644=AXIS2_PLACEMENT_3D ( 'NONE', #7998, #6931, #2662 ) ;
#11647=ORIENTED_EDGE ( 'NONE', *, *, #719, .T. ) ;
#11648=VECTOR ( 'NONE', #4351, 1000.000000000000000 ) ;
#11655=CYLINDRICAL_SURFACE ( 'NONE', #2670, 25.00000000000000711 ) ;
#11657=ORIENTED_EDGE ( 'NONE', *, *, #2870, .T. ) ;
#11663=EDGE_CURVE ( 'NONE', #6588, #13109, #2063, .T. ) ;
#11683=CARTESIAN_POINT ( 'NONE',  ( -24.99999999999998934, -100.0000000000000000, 7.500000000000000000 ) ) ;
#11698=ORIENTED_EDGE ( 'NONE', *, *, #6659, .T. ) ;
#11699=ORIENTED_EDGE ( 'NONE', *, *, #12884, .F. ) ;
#11709=DIRECTION ( 'NONE',  ( -0.000000000000000000, -0.000000000000000000, -1.000000000000000000 ) ) ;
#11718=EDGE_LOOP ( 'NONE', ( #2352, #11876, #9212, #12466, #1617, #10200, #8669, #10829, #12435, #2451 ) ) ;
#11720=CARTESIAN_POINT ( 'NONE',  ( 13.79311422413708499, -21.62638421600850691, -7.500000000000000000 ) ) ;
#11721=VERTEX_POINT ( 'NONE', #13364 ) ;
#11736=ORIENTED_EDGE ( 'NONE', *, *, #11180, .T. ) ;
#11742=AXIS2_PLACEMENT_3D ( 'NONE', #184, #1292, #8866 ) ;
#11746=AXIS2_PLACEMENT_3D ( 'NONE', #2130, #7393, #10485 ) ;
#11748=CARTESIAN_POINT ( 'NONE',  ( -35.00000000000000711, -25.00000000000000711, 7.500000000000000000 ) ) ;
#11751=FACE_OUTER_BOUND ( 'NONE', #6186, .T. ) ;
#11755=CIRCLE ( 'NONE', #799, 15.70031846811053455 ) ;
#11760=CARTESIAN_POINT ( 'NONE',  ( 19.18070798040252711, 20.00000000000000000, 4.000000000000000000 ) ) ;
#11770=ADVANCED_FACE ( 'NONE', ( #7766 ), #5744, .F. ) ;
#11772=ORIENTED_EDGE ( 'NONE', *, *, #13704, .F. ) ;
#11782=CARTESIAN_POINT ( 'NONE',  ( -35.00000000000000000, -35.00000000000000000, -7.500000000000000000 ) ) ;
#11788=ORIENTED_EDGE ( 'NONE', *, *, #1639, .T. ) ;
#11801=LINE ( 'NONE', #6478, #4235 ) ;
#11803=DIRECTION ( 'NONE',  ( -0.000000000000000000, 1.000000000000000000, -0.000000000000000000 ) ) ;
#11806=VERTEX_POINT ( 'NONE', #7926 ) ;
#11812=CARTESIAN_POINT ( 'NONE',  ( -18.54049621773915746, -20.00000000000000000, 7.500000000000000000 ) ) ;
#11815=CARTESIAN_POINT ( 'NONE',  ( -28.15981099771517648, -27.70535714287384366, 4.000000000000000000 ) ) ;
#11824=CARTESIAN_POINT ( 'NONE',  ( -35.00000000000000000, -4.286263797015736496E-15, -7.500000000000000000 ) ) ;
#11830=PLANE ( 'NONE',  #10273 ) ;
#11835=LINE ( 'NONE', #212, #12116 ) ;
#11838=DIRECTION ( 'NONE',  ( 0.000000000000000000, 0.000000000000000000, -1.000000000000000000 ) ) ;
#11845=DIRECTION ( 'NONE',  ( 0.000000000000000000, -0.000000000000000000, 1.000000000000000000 ) ) ;
#11847=CARTESIAN_POINT ( 'NONE',  ( 35.00000000000009237, 91.25000000000046896, -7.500000000000000000 ) ) ;
#11849=AXIS2_PLACEMENT_3D ( 'NONE', #10796, #1077, #9625 ) ;
#11866=DIRECTION ( 'NONE',  ( -1.000000000000000000, 0.000000000000000000, 0.000000000000000000 ) ) ;
#11869=DIRECTION ( 'NONE',  ( -1.224646799147353207E-16, 1.000000000000000000, -0.000000000000000000 ) ) ;
#11873=AXIS2_PLACEMENT_3D ( 'NONE', #2136, #5097, #6423 ) ;
#11876=ORIENTED_EDGE ( 'NONE', *, *, #13309, .T. ) ;
#11886=AXIS2_PLACEMENT_3D ( 'NONE', #9179, #2659, #5740 ) ;
#11895=EDGE_LOOP ( 'NONE', ( #9125, #2163, #9835, #7854, #12967, #4337, #5624, #12592, #265 ) ) ;
#11900=ORIENTED_EDGE ( 'NONE', *, *, #4625, .T. ) ;
#11901=EDGE_CURVE ( 'NONE', #9044, #10464, #3850, .T. ) ;
#11902=ORIENTED_EDGE ( 'NONE', *, *, #9530, .T. ) ;
#11903=EDGE_CURVE ( 'NONE', #13483, #5724, #4848, .T. ) ;
#11907=CARTESIAN_POINT ( 'NONE',  ( -60.00000000000001421, -4.286263797015736496E-15, 4.000000000000000000 ) ) ;
#11916=ORIENTED_EDGE ( 'NONE', *, *, #1458, .T. ) ;
#11920=EDGE_CURVE ( 'NONE', #11483, #13056, #774, .T. ) ;
#11927=DIRECTION ( 'NONE',  ( -0.000000000000000000, -0.000000000000000000, -1.000000000000000000 ) ) ;
#11928=CIRCLE ( 'NONE', #3411, 1.999999999999998224 ) ;
#11935=ADVANCED_FACE ( 'NONE', ( #5045 ), #10310, .F. ) ;
#11937=CYLINDRICAL_SURFACE ( 'NONE', #6279, 2.500000000000002220 ) ;
#11938=CARTESIAN_POINT ( 'NONE',  ( 34.99999999999999289, 25.00000000000002132, 4.000000000000000000 ) ) ;
#11941=CARTESIAN_POINT ( 'NONE',  ( 31.93204061526060045, 3.910547132972217398E-15, 3.910547132972217398E-15 ) ) ;
#11951=CARTESIAN_POINT ( 'NONE',  ( -35.00000000000000000, -35.00000000000000000, -4.000000000000000000 ) ) ;
#11969=ORIENTED_EDGE ( 'NONE', *, *, #7775, .F. ) ;
#11980=PLANE ( 'NONE',  #13003 ) ;
#11981=CARTESIAN_POINT ( 'NONE',  ( 35.00000000000000000, -4.286263797015736496E-15, -4.000000000000000000 ) ) ;
#11989=TOROIDAL_SURFACE ( 'NONE', #6183, -34.24999999999974420, 69.24999999999975842 ) ;
#11990=DIRECTION ( 'NONE',  ( -1.000000000000000000, 0.000000000000000000, 0.000000000000000000 ) ) ;
#11996=DIRECTION ( 'NONE',  ( 0.000000000000000000, 0.000000000000000000, 1.000000000000000000 ) ) ;
#11999=LINE ( 'NONE', #98, #11648 ) ;
#12001=EDGE_CURVE ( 'NONE', #4125, #5724, #8524, .T. ) ;
#12002=CARTESIAN_POINT ( 'NONE',  ( 32.50000000000000000, 4.286263797015736496E-15, -4.000000000000000000 ) ) ;
#12006=ADVANCED_FACE ( 'NONE', ( #261 ), #4377, .F. ) ;
#12009=DIRECTION ( 'NONE',  ( 0.000000000000000000, 0.000000000000000000, 1.000000000000000000 ) ) ;
#12013=CARTESIAN_POINT ( 'NONE',  ( -23.64268088454699779, -97.00000000000000000, 0.000000000000000000 ) ) ;
#12014=FACE_OUTER_BOUND ( 'NONE', #2046, .T. ) ;
#12015=EDGE_LOOP ( 'NONE', ( #12879, #4556, #6897, #10949 ) ) ;
#12078=VECTOR ( 'NONE', #13410, 1000.000000000000000 ) ;
#12087=ORIENTED_EDGE ( 'NONE', *, *, #8399, .T. ) ;
#12097=CARTESIAN_POINT ( 'NONE',  ( 35.00000000000000000, -4.286263797015736496E-15, 4.000000000000000000 ) ) ;
#12113=ORIENTED_EDGE ( 'NONE', *, *, #8153, .F. ) ;
#12116=VECTOR ( 'NONE', #6376, 1000.000000000000000 ) ;
#12121=SURFACE_STYLE_USAGE ( .BOTH. , #2514 ) ;
#12122=ORIENTED_EDGE ( 'NONE', *, *, #11663, .T. ) ;
#12124=VECTOR ( 'NONE', #2838, 1000.000000000000000 ) ;
#12133=CARTESIAN_POINT ( 'NONE',  ( 19.38529118556630237, 26.86594603178324903, -5.082853661574512572 ) ) ;
#12144=ORIENTED_EDGE ( 'NONE', *, *, #10365, .T. ) ;
#12148=PLANE ( 'NONE',  #13888 ) ;
#12153=EDGE_LOOP ( 'NONE', ( #3856, #13159, #11212, #5569 ) ) ;
#12162=VERTEX_POINT ( 'NONE', #2843 ) ;
#12169=CARTESIAN_POINT ( 'NONE',  ( 26.79177319725820539, -26.24642857144861807, 4.000000000000000000 ) ) ;
#12173=EDGE_CURVE ( 'NONE', #9444, #10078, #11390, .T. ) ;
#12178=ORIENTED_EDGE ( 'NONE', *, *, #1082, .T. ) ;
#12181=ORIENTED_EDGE ( 'NONE', *, *, #10772, .F. ) ;
#12188=DIRECTION ( 'NONE',  ( 0.000000000000000000, 0.000000000000000000, -1.000000000000000000 ) ) ;
#12193=EDGE_CURVE ( 'NONE', #8713, #12944, #2550, .T. ) ;
#12196=EDGE_CURVE ( 'NONE', #12494, #1107, #7687, .T. ) ;
#12203=DIRECTION ( 'NONE',  ( -1.000000000000000000, 0.000000000000000000, 0.000000000000000000 ) ) ;
#12207=CIRCLE ( 'NONE', #13829, 20.00000000000000000 ) ;
#12214=ORIENTED_EDGE ( 'NONE', *, *, #12957, .T. ) ;
#12218=LINE ( 'NONE', #10245, #13108 ) ;
#12227=DIRECTION ( 'NONE',  ( -1.000000000000000000, -1.224646799147353207E-16, 0.000000000000000000 ) ) ;
#12228=CARTESIAN_POINT ( 'NONE',  ( 15.47908363509431595, -16.40738050097609602, 2.711248065311635091 ) ) ;
#12229=( GEOMETRIC_REPRESENTATION_CONTEXT ( 3 ) GLOBAL_UNCERTAINTY_ASSIGNED_CONTEXT ( ( #4763 ) ) GLOBAL_UNIT_ASSIGNED_CONTEXT ( ( #7860, #1207, #4491 ) ) REPRESENTATION_CONTEXT ( 'NONE', 'WORKASPACE' ) );
#12231=ORIENTED_EDGE ( 'NONE', *, *, #7825, .T. ) ;
#12233=DIRECTION ( 'NONE',  ( -1.000000000000000000, 0.000000000000000000, 0.000000000000000000 ) ) ;
#12245=DIRECTION ( 'NONE',  ( 1.000000000000000000, 0.000000000000000000, 1.224646799147352961E-16 ) ) ;
#12246=DIRECTION ( 'NONE',  ( 0.000000000000000000, 1.000000000000000000, 0.000000000000000000 ) ) ;
#12253=ORIENTED_EDGE ( 'NONE', *, *, #2304, .T. ) ;
#12258=CARTESIAN_POINT ( 'NONE',  ( 0.000000000000000000, -20.00000000000000000, 0.000000000000000000 ) ) ;
#12264=EDGE_LOOP ( 'NONE', ( #6729, #2250, #8275, #10945 ) ) ;
#12265=ORIENTED_EDGE ( 'NONE', *, *, #966, .F. ) ;
#12266=ADVANCED_FACE ( 'NONE', ( #8443 ), #12731, .F. ) ;
#12279=EDGE_LOOP ( 'NONE', ( #4112, #4836, #11001, #6010, #3992, #22, #12576, #2264, #3857, #7029 ) ) ;
#12296=DIRECTION ( 'NONE',  ( 0.000000000000000000, 1.000000000000000000, 0.000000000000000000 ) ) ;
#12301=ORIENTED_EDGE ( 'NONE', *, *, #2304, .F. ) ;
#12313=DIRECTION ( 'NONE',  ( 0.000000000000000000, 0.000000000000000000, 1.000000000000000000 ) ) ;
#12314=FACE_OUTER_BOUND ( 'NONE', #2314, .T. ) ;
#12325=AXIS2_PLACEMENT_3D ( 'NONE', #5286, #13682, #8377 ) ;
#12337=AXIS2_PLACEMENT_3D ( 'NONE', #7662, #4505, #10810 ) ;
#12341=EDGE_LOOP ( 'NONE', ( #7657, #4319 ) ) ;
#12348=FACE_OUTER_BOUND ( 'NONE', #9111, .T. ) ;
#12351=DIRECTION ( 'NONE',  ( 0.000000000000000000, 0.000000000000000000, 1.000000000000000000 ) ) ;
#12354=VECTOR ( 'NONE', #7518, 1000.000000000000000 ) ;
#12357=AXIS2_PLACEMENT_3D ( 'NONE', #3003, #8400, #7073 ) ;
#12360=ORIENTED_EDGE ( 'NONE', *, *, #9620, .T. ) ;
#12369=DIRECTION ( 'NONE',  ( 0.000000000000000000, 0.000000000000000000, 1.000000000000000000 ) ) ;
#12371=DIRECTION ( 'NONE',  ( -0.000000000000000000, -0.000000000000000000, -1.000000000000000000 ) ) ;
#12374=ORIENTED_EDGE ( 'NONE', *, *, #10624, .F. ) ;
#12376=CARTESIAN_POINT ( 'NONE',  ( -6.999999999999999112, -35.00000000000000000, 7.500000000000000000 ) ) ;
#12382=FACE_BOUND ( 'NONE', #12763, .T. ) ;
#12392=CARTESIAN_POINT ( 'NONE',  ( -19.51309799441515125, 26.83545189264576791, -4.432601239563245699 ) ) ;
#12394=ADVANCED_FACE ( 'NONE', ( #4567, #13089 ), #2262, .T. ) ;
#12402=CARTESIAN_POINT ( 'NONE',  ( -15.70039857998626864, -16.66659488452782156, 0.6827713257413515757 ) ) ;
#12405=CARTESIAN_POINT ( 'NONE',  ( -35.00000000000000000, -4.286263797015736496E-15, 7.500000000000000000 ) ) ;
#12409=VERTEX_POINT ( 'NONE', #9634 ) ;
#12412=VERTEX_POINT ( 'NONE', #5481 ) ;
#12420=ORIENTED_EDGE ( 'NONE', *, *, #6621, .F. ) ;
#12430=CARTESIAN_POINT ( 'NONE',  ( 35.00000000000000000, 4.286263797015736496E-15, 4.000000000000000000 ) ) ;
#12431=CARTESIAN_POINT ( 'NONE',  ( 15.48128881649354405, -16.40999965198128052, -2.699219240941213460 ) ) ;
#12435=ORIENTED_EDGE ( 'NONE', *, *, #1465, .T. ) ;
#12442=CARTESIAN_POINT ( 'NONE',  ( -26.79177319725820894, -26.24642857144861807, 4.000000000000000000 ) ) ;
#12444=ORIENTED_EDGE ( 'NONE', *, *, #12471, .F. ) ;
#12445=CIRCLE ( 'NONE', #9748, 2.000000000000001776 ) ;
#12453=DIRECTION ( 'NONE',  ( -1.000000000000000000, 0.000000000000000000, 0.000000000000000000 ) ) ;
#12466=ORIENTED_EDGE ( 'NONE', *, *, #11093, .F. ) ;
#12471=EDGE_CURVE ( 'NONE', #2423, #4467, #1423, .T. ) ;
#12472=DIRECTION ( 'NONE',  ( 0.000000000000000000, 0.000000000000000000, 1.000000000000000000 ) ) ;
#12477=ORIENTED_EDGE ( 'NONE', *, *, #5306, .F. ) ;
#12481=EDGE_LOOP ( 'NONE', ( #2267, #11916, #3067 ) ) ;
#12489=DIRECTION ( 'NONE',  ( 0.000000000000000000, 1.000000000000000000, 0.000000000000000000 ) ) ;
#12494=VERTEX_POINT ( 'NONE', #11170 ) ;
#12507=CARTESIAN_POINT ( 'NONE',  ( 22.00000000000000355, -34.99999999999999289, -7.500000000000000000 ) ) ;
#12508=EDGE_LOOP ( 'NONE', ( #13881, #1767, #2157, #1138, #665, #3878, #8416, #5049 ) ) ;
#12510=EDGE_CURVE ( 'NONE', #8361, #7055, #13342, .T. ) ;
#12517=DIRECTION ( 'NONE',  ( -0.000000000000000000, -0.000000000000000000, -1.000000000000000000 ) ) ;
#12537=VERTEX_POINT ( 'NONE', #9137 ) ;
#12541=CYLINDRICAL_SURFACE ( 'NONE', #8811, 25.00000000000000711 ) ;
#12543=CARTESIAN_POINT ( 'NONE',  ( 15.37190086779362908, -22.55217709030014817, -3.259922557882396710 ) ) ;
#12555=CIRCLE ( 'NONE', #7161, 2.500000000000002220 ) ;
#12559=DIRECTION ( 'NONE',  ( -0.000000000000000000, -0.000000000000000000, -1.000000000000000000 ) ) ;
#12565=ADVANCED_FACE ( 'NONE', ( #457 ), #11989, .T. ) ;
#12576=ORIENTED_EDGE ( 'NONE', *, *, #309, .T. ) ;
#12583=DIRECTION ( 'NONE',  ( 0.000000000000000000, 0.000000000000000000, 1.000000000000000000 ) ) ;
#12584=VECTOR ( 'NONE', #4932, 1000.000000000000000 ) ;
#12590=CIRCLE ( 'NONE', #6308, 2.000000000000001776 ) ;
#12592=ORIENTED_EDGE ( 'NONE', *, *, #5771, .T. ) ;
#12593=CARTESIAN_POINT ( 'NONE',  ( 34.99999999999999289, 25.00000000000002132, 7.500000000000000000 ) ) ;
#12599=CARTESIAN_POINT ( 'NONE',  ( 7.000000000000007994, -35.00000000000000000, -7.500000000000000000 ) ) ;
#12601=CIRCLE ( 'NONE', #280, 25.00000000000000355 ) ;
#12602=B_SPLINE_CURVE_WITH_KNOTS ( 'NONE', 3,
 ( #8605, #5374, #1182, #6711 ),
 .UNSPECIFIED., .F., .F.,
 ( 4, 4 ),
 ( 0.03713967652845534539, 0.04074225392669957035 ),
 .UNSPECIFIED. ) ;
#12604=DIRECTION ( 'NONE',  ( -0.000000000000000000, -0.000000000000000000, -1.000000000000000000 ) ) ;
#12609=DIRECTION ( 'NONE',  ( 0.000000000000000000, 0.000000000000000000, 1.000000000000000000 ) ) ;
#12611=EDGE_CURVE ( 'NONE', #12961, #3769, #11099, .T. ) ;
#12612=CARTESIAN_POINT ( 'NONE',  ( 15.04986406078724848, -22.34153611474686230, -4.519294538364309943 ) ) ;
#12618=LINE ( 'NONE', #7201, #3642 ) ;
#12619=LINE ( 'NONE', #7268, #9161 ) ;
#12625=ORIENTED_EDGE ( 'NONE', *, *, #7825, .F. ) ;
#12631=EDGE_CURVE ( 'NONE', #4480, #11806, #2595, .T. ) ;
#12640=CARTESIAN_POINT ( 'NONE',  ( -35.00000000000000000, -4.286263797015736496E-15, 7.500000000000000000 ) ) ;
#12641=EDGE_CURVE ( 'NONE', #13124, #1407, #3045, .T. ) ;
#12643=VERTEX_POINT ( 'NONE', #12507 ) ;
#12649=CYLINDRICAL_SURFACE ( 'NONE', #3389, 22.00000000000000000 ) ;
#12650=DIRECTION ( 'NONE',  ( -1.601283208593975514E-16, 1.000000000000000000, -0.000000000000000000 ) ) ;
#12652=DIRECTION ( 'NONE',  ( -0.000000000000000000, -0.000000000000000000, -1.000000000000000000 ) ) ;
#12664=CIRCLE ( 'NONE', #11742, 66.25000000000044054 ) ;
#12668=AXIS2_PLACEMENT_3D ( 'NONE', #742, #12517, #5007 ) ;
#12670=DIRECTION ( 'NONE',  ( 0.000000000000000000, 0.000000000000000000, 1.000000000000000000 ) ) ;
#12672=LINE ( 'NONE', #11603, #6712 ) ;
#12677=DIRECTION ( 'NONE',  ( 1.000000000000000000, -0.000000000000000000, -0.000000000000000000 ) ) ;
#12689=AXIS2_PLACEMENT_3D ( 'NONE', #2872, #8133, #7146 ) ;
#12696=CARTESIAN_POINT ( 'NONE',  ( -15.18222645069203303, -16.04698886238941924, -4.000000000000000000 ) ) ;
#12698=ORIENTED_EDGE ( 'NONE', *, *, #1082, .F. ) ;
#12701=EDGE_CURVE ( 'NONE', #9446, #12162, #6850, .T. ) ;
#12708=CARTESIAN_POINT ( 'NONE',  ( 35.00000000000001421, -34.99999999999999289, -4.000000000000000000 ) ) ;
#12714=LINE ( 'NONE', #2841, #9927 ) ;
#12717=ORIENTED_EDGE ( 'NONE', *, *, #1214, .F. ) ;
#12718=VERTEX_POINT ( 'NONE', #1765 ) ;
#12731=CYLINDRICAL_SURFACE ( 'NONE', #4113, 25.50000000002550138 ) ;
#12736=EDGE_LOOP ( 'NONE', ( #9725, #7459, #2024, #1343, #1962, #5811 ) ) ;
#12741=FACE_OUTER_BOUND ( 'NONE', #13523, .T. ) ;
#12757=DIRECTION ( 'NONE',  ( 1.000000000000000000, 0.000000000000000000, 0.000000000000000000 ) ) ;
#12760=CIRCLE ( 'NONE', #11199, 25.50418395392908977 ) ;
#12761=( NAMED_UNIT ( * ) PLANE_ANGLE_UNIT ( ) SI_UNIT ( $, .RADIAN. ) );
#12763=EDGE_LOOP ( 'NONE', ( #1140, #10095 ) ) ;
#12764=ORIENTED_EDGE ( 'NONE', *, *, #8799, .T. ) ;
#12766=DIRECTION ( 'NONE',  ( 0.000000000000000000, 0.000000000000000000, 1.000000000000000000 ) ) ;
#12774=ORIENTED_EDGE ( 'NONE', *, *, #13181, .T. ) ;
#12776=ADVANCED_FACE ( 'NONE', ( #2241, #2305 ), #6526, .T. ) ;
#12780=CARTESIAN_POINT ( 'NONE',  ( -24.99999999999999289, -99.43893449056518818, 2.967955073073089700 ) ) ;
#12782=VECTOR ( 'NONE', #8285, 1000.000000000000000 ) ;
#12788=VERTEX_POINT ( 'NONE', #82 ) ;
#12791=CARTESIAN_POINT ( 'NONE',  ( 1.616533774874506480E-14, -132.0000000000000000, 0.000000000000000000 ) ) ;
#12795=CIRCLE ( 'NONE', #7852, 31.93204061526060755 ) ;
#12820=DIRECTION ( 'NONE',  ( -1.000000000000000000, 0.000000000000000000, 0.000000000000000000 ) ) ;
#12823=LINE ( 'NONE', #8387, #2317 ) ;
#12827=CARTESIAN_POINT ( 'NONE',  ( -32.50000000000000000, -3.980102097228898626E-15, 7.500000000000000000 ) ) ;
#12828=EDGE_CURVE ( 'NONE', #11308, #4855, #7565, .T. ) ;
#12843=ORIENTED_EDGE ( 'NONE', *, *, #6340, .T. ) ;
#12851=CARTESIAN_POINT ( 'NONE',  ( -27.38873514654796537, -24.33759740261776017, 4.000000000000000000 ) ) ;
#12855=VECTOR ( 'NONE', #3559, 1000.000000000000000 ) ;
#12861=EDGE_CURVE ( 'NONE', #6130, #5016, #1922, .T. ) ;
#12879=ORIENTED_EDGE ( 'NONE', *, *, #2781, .F. ) ;
#12881=ORIENTED_EDGE ( 'NONE', *, *, #3548, .F. ) ;
#12884=EDGE_CURVE ( 'NONE', #1355, #1592, #1134, .T. ) ;
#12899=AXIS2_PLACEMENT_3D ( 'NONE', #8381, #3053, #9774 ) ;
#12906=CARTESIAN_POINT ( 'NONE',  ( 25.00000000000000711, -99.51472204732195337, 3.411167378945609840 ) ) ;
#12914=VECTOR ( 'NONE', #1839, 1000.000000000000000 ) ;
#12918=EDGE_LOOP ( 'NONE', ( #13703, #12144, #10506 ) ) ;
#12921=LINE ( 'NONE', #7557, #6074 ) ;
#12929=ORIENTED_EDGE ( 'NONE', *, *, #1891, .T. ) ;
#12944=VERTEX_POINT ( 'NONE', #1399 ) ;
#12945=CARTESIAN_POINT ( 'NONE',  ( -35.00000000000000000, -4.286263797015736496E-15, 7.500000000000000000 ) ) ;
#12947=CARTESIAN_POINT ( 'NONE',  ( -24.99999999999998934, -99.15310334213020838, 4.530792947966844994E-20 ) ) ;
#12951=ORIENTED_EDGE ( 'NONE', *, *, #4138, .F. ) ;
#12957=EDGE_CURVE ( 'NONE', #2827, #12412, #7769, .T. ) ;
#12961=VERTEX_POINT ( 'NONE', #13134 ) ;
#12967=ORIENTED_EDGE ( 'NONE', *, *, #10971, .T. ) ;
#12974=DIRECTION ( 'NONE',  ( 1.000000000000000000, 0.000000000000000000, 0.000000000000000000 ) ) ;
#12977=ORIENTED_EDGE ( 'NONE', *, *, #1968, .T. ) ;
#12979=ORIENTED_EDGE ( 'NONE', *, *, #6430, .F. ) ;
#12984=LINE ( 'NONE', #75, #3626 ) ;
#12987=FACE_OUTER_BOUND ( 'NONE', #12264, .T. ) ;
#13003=AXIS2_PLACEMENT_3D ( 'NONE', #2299, #9674, #3149 ) ;
#13014=AXIS2_PLACEMENT_3D ( 'NONE', #12599, #4089, #39 ) ;
#13018=PLANE ( 'NONE',  #3470 ) ;
#13022=ORIENTED_EDGE ( 'NONE', *, *, #4114, .T. ) ;
#13030=DIRECTION ( 'NONE',  ( -0.000000000000000000, -0.000000000000000000, -1.000000000000000000 ) ) ;
#13044=CARTESIAN_POINT ( 'NONE',  ( 18.54049621773915746, -20.00000000000000000, 7.500000000000000000 ) ) ;
#13056=VERTEX_POINT ( 'NONE', #10541 ) ;
#13070=EDGE_LOOP ( 'NONE', ( #13022, #6456, #2652, #11536 ) ) ;
#13071=ORIENTED_EDGE ( 'NONE', *, *, #12193, .T. ) ;
#13077=DIRECTION ( 'NONE',  ( -1.000000000000000000, -1.224646799147353207E-16, 0.000000000000000000 ) ) ;
#13078=SHAPE_REPRESENTATION_RELATIONSHIP ( 'NONE' , 'NONE' ,  #2342, #11412 ) ;
#13084=FACE_OUTER_BOUND ( 'NONE', #7730, .T. ) ;
#13089=FACE_OUTER_BOUND ( 'NONE', #10662, .T. ) ;
#13095=CARTESIAN_POINT ( 'NONE',  ( 15.18222645069203125, -100.0000000000000000, -4.000000000000000000 ) ) ;
#13106=EDGE_LOOP ( 'NONE', ( #3966, #7913 ) ) ;
#13108=VECTOR ( 'NONE', #2531, 1000.000000000000000 ) ;
#13109=VERTEX_POINT ( 'NONE', #2322 ) ;
#13113=AXIS2_PLACEMENT_3D ( 'NONE', #10486, #10558, #12820 ) ;
#13114=CARTESIAN_POINT ( 'NONE',  ( -35.00000000000000000, -4.286263797015736496E-15, 7.500000000000000000 ) ) ;
#13122=LINE ( 'NONE', #4537, #697 ) ;
#13124=VERTEX_POINT ( 'NONE', #12002 ) ;
#13134=CARTESIAN_POINT ( 'NONE',  ( -21.99999999999997868, -100.0000000000000000, 0.000000000000000000 ) ) ;
#13140=VECTOR ( 'NONE', #8826, 1000.000000000000000 ) ;
#13141=EDGE_CURVE ( 'NONE', #2577, #6733, #12207, .T. ) ;
#13157=DIRECTION ( 'NONE',  ( 0.000000000000000000, -0.000000000000000000, 1.000000000000000000 ) ) ;
#13159=ORIENTED_EDGE ( 'NONE', *, *, #2094, .T. ) ;
#13165=ORIENTED_EDGE ( 'NONE', *, *, #6701, .T. ) ;
#13168=DIRECTION ( 'NONE',  ( -1.000000000000000000, 0.000000000000000000, 0.000000000000000000 ) ) ;
#13181=EDGE_CURVE ( 'NONE', #7055, #3625, #9375, .T. ) ;
#13189=CARTESIAN_POINT ( 'NONE',  ( 35.00000000000009237, 91.25000000000046896, -4.000000000000000000 ) ) ;
#13206=DIRECTION ( 'NONE',  ( 0.000000000000000000, -0.000000000000000000, 1.000000000000000000 ) ) ;
#13210=CIRCLE ( 'NONE', #1097, 25.50000000002550138 ) ;
#13229=FACE_OUTER_BOUND ( 'NONE', #9025, .T. ) ;
#13235=VECTOR ( 'NONE', #2695, 1000.000000000000000 ) ;
#13237=CARTESIAN_POINT ( 'NONE',  ( 30.72062512117245703, 25.13835616439070719, 4.000000000000000000 ) ) ;
#13239=CARTESIAN_POINT ( 'NONE',  ( -34.24999999999972999, -135.0000000000000000, -4.194415287079653581E-15 ) ) ;
#13248=DIRECTION ( 'NONE',  ( -0.000000000000000000, 1.000000000000000000, -0.000000000000000000 ) ) ;
#13249=VECTOR ( 'NONE', #181, 1000.000000000000000 ) ;
#13253=DIRECTION ( 'NONE',  ( -0.000000000000000000, -0.000000000000000000, -1.000000000000000000 ) ) ;
#13263=CIRCLE ( 'NONE', #6731, 25.00000000000000711 ) ;
#13269=DIRECTION ( 'NONE',  ( -0.000000000000000000, -0.000000000000000000, -1.000000000000000000 ) ) ;
#13271=ORIENTED_EDGE ( 'NONE', *, *, #1742, .F. ) ;
#13273=ADVANCED_FACE ( 'NONE', ( #9573 ), #6223, .F. ) ;
#13278=FILL_AREA_STYLE_COLOUR ( '', #2277 ) ;
#13281=VECTOR ( 'NONE', #6411, 1000.000000000000000 ) ;
#13289=EDGE_LOOP ( 'NONE', ( #12698, #2557, #5681, #6222 ) ) ;
#13305=CARTESIAN_POINT ( 'NONE',  ( -35.00000000000000000, -4.286263797015736496E-15, -4.000000000000000000 ) ) ;
#13306=CARTESIAN_POINT ( 'NONE',  ( 1.387778780781445676E-14, -135.0000000000000000, 0.000000000000000000 ) ) ;
#13307=EDGE_LOOP ( 'NONE', ( #6095, #8802, #3066, #9658 ) ) ;
#13309=EDGE_CURVE ( 'NONE', #2284, #12537, #2197, .T. ) ;
#13316=AXIS2_PLACEMENT_3D ( 'NONE', #3622, #7830, #5955 ) ;
#13326=DIRECTION ( 'NONE',  ( -1.000000000000000000, 0.000000000000000000, 0.000000000000000000 ) ) ;
#13332=EDGE_CURVE ( 'NONE', #12944, #12643, #8518, .T. ) ;
#13337=ORIENTED_EDGE ( 'NONE', *, *, #10210, .F. ) ;
#13342=CIRCLE ( 'NONE', #7250, 20.00000000000000000 ) ;
#13354=AXIS2_PLACEMENT_3D ( 'NONE', #13189, #13269, #7903 ) ;
#13359=ORIENTED_EDGE ( 'NONE', *, *, #8828, .F. ) ;
#13363=DIRECTION ( 'NONE',  ( 0.000000000000000000, 0.000000000000000000, 1.000000000000000000 ) ) ;
#13364=CARTESIAN_POINT ( 'NONE',  ( 1.922734475756564121E-15, -20.00000000000000355, -15.70031846811053455 ) ) ;
#13370=CIRCLE ( 'NONE', #12899, 25.00000000000000711 ) ;
#13377=DIRECTION ( 'NONE',  ( 1.000000000000000000, -0.000000000000000000, -0.000000000000000000 ) ) ;
#13382=DIRECTION ( 'NONE',  ( -0.000000000000000000, -0.000000000000000000, -1.000000000000000000 ) ) ;
#13383=AXIS2_PLACEMENT_3D ( 'NONE', #9906, #595, #12227 ) ;
#13392=VERTEX_POINT ( 'NONE', #1093 ) ;
#13398=EDGE_LOOP ( 'NONE', ( #4987, #8761, #8195, #9349, #10166, #10201, #230, #1573, #10174 ) ) ;
#13404=CARTESIAN_POINT ( 'NONE',  ( 0.000000000000000000, -20.00000000000000000, 0.000000000000000000 ) ) ;
#13410=DIRECTION ( 'NONE',  ( -0.000000000000000000, -0.000000000000000000, -1.000000000000000000 ) ) ;
#13422=LINE ( 'NONE', #5885, #7315 ) ;
#13446=ORIENTED_EDGE ( 'NONE', *, *, #11266, .T. ) ;
#13450=DIRECTION ( 'NONE',  ( 0.000000000000000000, 0.000000000000000000, 1.000000000000000000 ) ) ;
#13456=DIRECTION ( 'NONE',  ( -1.224646799147353207E-16, 1.000000000000000000, -0.000000000000000000 ) ) ;
#13457=ORIENTED_EDGE ( 'NONE', *, *, #3241, .F. ) ;
#13461=LINE ( 'NONE', #535, #2256 ) ;
#13465=DIRECTION ( 'NONE',  ( 1.000000000000000000, 0.000000000000000000, 1.224646799147353207E-16 ) ) ;
#13472=TOROIDAL_SURFACE ( 'NONE', #11849, -34.24999999999974420, 66.24999999999978684 ) ;
#13483=VERTEX_POINT ( 'NONE', #9844 ) ;
#13486=AXIS2_PLACEMENT_3D ( 'NONE', #13239, #9987, #13465 ) ;
#13489=CARTESIAN_POINT ( 'NONE',  ( -15.68886946032145957, -16.65327071804363612, -0.6902218057983463551 ) ) ;
#13498=ORIENTED_EDGE ( 'NONE', *, *, #1214, .T. ) ;
#13507=CARTESIAN_POINT ( 'NONE',  ( 13.79311422413708499, -100.0000000000000000, -7.500000000000000000 ) ) ;
#13515=AXIS2_PLACEMENT_3D ( 'NONE', #10052, #8934, #8159 ) ;
#13521=DIRECTION ( 'NONE',  ( -1.000000000000000000, 0.000000000000000000, 0.000000000000000000 ) ) ;
#13523=EDGE_LOOP ( 'NONE', ( #3476, #11362, #11736, #3478, #3554, #7334, #5187, #5975, #10719, #607, #10499, #8852, #11554 ) ) ;
#13528=CARTESIAN_POINT ( 'NONE',  ( 28.15981099771517648, -27.70535714287384366, -4.000000000000000000 ) ) ;
#13530=ORIENTED_EDGE ( 'NONE', *, *, #7135, .F. ) ;
#13537=CARTESIAN_POINT ( 'NONE',  ( 18.54049621773915746, 27.07720798312000809, 7.500000000000000000 ) ) ;
#13541=CYLINDRICAL_SURFACE ( 'NONE', #11630, 10.00000000000000178 ) ;
#13575=VECTOR ( 'NONE', #5580, 1000.000000000000000 ) ;
#13578=CARTESIAN_POINT ( 'NONE',  ( 1.387778780781445676E-14, -135.0000000000000000, 0.000000000000000000 ) ) ;
#13581=VERTEX_POINT ( 'NONE', #4507 ) ;
#13585=ADVANCED_FACE ( 'NONE', ( #1500 ), #9918, .F. ) ;
#13594=ORIENTED_EDGE ( 'NONE', *, *, #13689, .T. ) ;
#13596=ORIENTED_EDGE ( 'NONE', *, *, #2561, .F. ) ;
#13603=EDGE_CURVE ( 'NONE', #10943, #7680, #11755, .T. ) ;
#13615=AXIS2_PLACEMENT_3D ( 'NONE', #11981, #10100, #9957 ) ;
#13630=EDGE_CURVE ( 'NONE', #4098, #12961, #9304, .T. ) ;
#13633=CIRCLE ( 'NONE', #9338, 25.00000000000000355 ) ;
#13635=EDGE_LOOP ( 'NONE', ( #12265, #6757, #5268, #3078 ) ) ;
#13646=VERTEX_POINT ( 'NONE', #13537 ) ;
#13652=DIRECTION ( 'NONE',  ( -1.000000000000000000, 0.000000000000000000, 0.000000000000000000 ) ) ;
#13655=CARTESIAN_POINT ( 'NONE',  ( -15.69972745459287822, -22.78055882083340222, -0.6693078754302107525 ) ) ;
#13673=DIRECTION ( 'NONE',  ( -0.000000000000000000, -0.000000000000000000, -1.000000000000000000 ) ) ;
#13676=DIRECTION ( 'NONE',  ( 0.000000000000000000, 0.000000000000000000, 1.000000000000000000 ) ) ;
#13678=AXIS2_PLACEMENT_3D ( 'NONE', #9544, #13726, #7428 ) ;
#13681=ORIENTED_EDGE ( 'NONE', *, *, #12641, .F. ) ;
#13682=DIRECTION ( 'NONE',  ( 0.000000000000000000, 1.000000000000000000, 0.000000000000000000 ) ) ;
#13688=AXIS2_PLACEMENT_3D ( 'NONE', #10864, #1151, #11996 ) ;
#13689=EDGE_CURVE ( 'NONE', #1355, #6722, #8611, .T. ) ;
#13700=VECTOR ( 'NONE', #11927, 1000.000000000000000 ) ;
#13703=ORIENTED_EDGE ( 'NONE', *, *, #9527, .F. ) ;
#13704=EDGE_CURVE ( 'NONE', #1407, #7751, #2901, .T. ) ;
#13710=VECTOR ( 'NONE', #4264, 1000.000000000000000 ) ;
#13714=DIRECTION ( 'NONE',  ( -1.000000000000000000, 0.000000000000000000, 0.000000000000000000 ) ) ;
#13717=AXIS2_PLACEMENT_3D ( 'NONE', #3120, #8522, #1873 ) ;
#13721=ORIENTED_EDGE ( 'NONE', *, *, #13765, .F. ) ;
#13726=DIRECTION ( 'NONE',  ( 0.000000000000000000, 0.000000000000000000, 1.000000000000000000 ) ) ;
#13746=AXIS2_PLACEMENT_3D ( 'NONE', #4563, #13382, #3732 ) ;
#13752=CARTESIAN_POINT ( 'NONE',  ( 15.18222645069203303, 20.00000000000000000, -4.000000000000000000 ) ) ;
#13753=ORIENTED_EDGE ( 'NONE', *, *, #8067, .T. ) ;
#13756=CARTESIAN_POINT ( 'NONE',  ( 14.37641089434894326, -21.93614314624078787, -6.343488216808988334 ) ) ;
#13764=EDGE_CURVE ( 'NONE', #9113, #11308, #6394, .T. ) ;
#13765=EDGE_CURVE ( 'NONE', #2392, #6130, #11258, .T. ) ;
#13771=CARTESIAN_POINT ( 'NONE',  ( -21.99999999999999289, -97.00000000000000000, 7.500000000000000000 ) ) ;
#13776=CARTESIAN_POINT ( 'NONE',  ( 13.79311422413708499, -21.62638421600850691, 7.500000000000000000 ) ) ;
#13781=ORIENTED_EDGE ( 'NONE', *, *, #3614, .F. ) ;
#13782=DIRECTION ( 'NONE',  ( -1.000000000000000000, 0.000000000000000000, 0.000000000000000000 ) ) ;
#13788=CARTESIAN_POINT ( 'NONE',  ( -15.37190086779363263, -22.55217709030015527, 3.259922557882396710 ) ) ;
#13797=ORIENTED_EDGE ( 'NONE', *, *, #7609, .F. ) ;
#13799=DIRECTION ( 'NONE',  ( -1.224646799147353207E-16, 1.000000000000000000, -0.000000000000000000 ) ) ;
#13803=CIRCLE ( 'NONE', #9068, 2.500000000000002220 ) ;
#13811=DIRECTION ( 'NONE',  ( 1.000000000000000000, 0.000000000000000000, 0.000000000000000000 ) ) ;
#13812=LINE ( 'NONE', #9502, #9181 ) ;
#13814=VECTOR ( 'NONE', #2331, 1000.000000000000000 ) ;
#13829=AXIS2_PLACEMENT_3D ( 'NONE', #11399, #2851, #12609 ) ;
#13839=FACE_OUTER_BOUND ( 'NONE', #7954, .T. ) ;
#13855=CARTESIAN_POINT ( 'NONE',  ( -14.10210168181666113, -21.78333407367943053, 6.931746760319975387 ) ) ;
#13857=DIRECTION ( 'NONE',  ( 0.000000000000000000, 0.000000000000000000, 1.000000000000000000 ) ) ;
#13878=FACE_OUTER_BOUND ( 'NONE', #7291, .T. ) ;
#13879=VERTEX_POINT ( 'NONE', #4635 ) ;
#13881=ORIENTED_EDGE ( 'NONE', *, *, #10211, .F. ) ;
#13885=DIRECTION ( 'NONE',  ( -1.000000000000000000, 0.000000000000000000, 0.000000000000000000 ) ) ;
#13888=AXIS2_PLACEMENT_3D ( 'NONE', #2320, #2257, #10798 ) ;
#13889=CARTESIAN_POINT ( 'NONE',  ( -18.54049621773915746, 27.07720798311999388, 7.500000000000000000 ) ) ;
ENDSEC;
END-ISO-10303-21;
